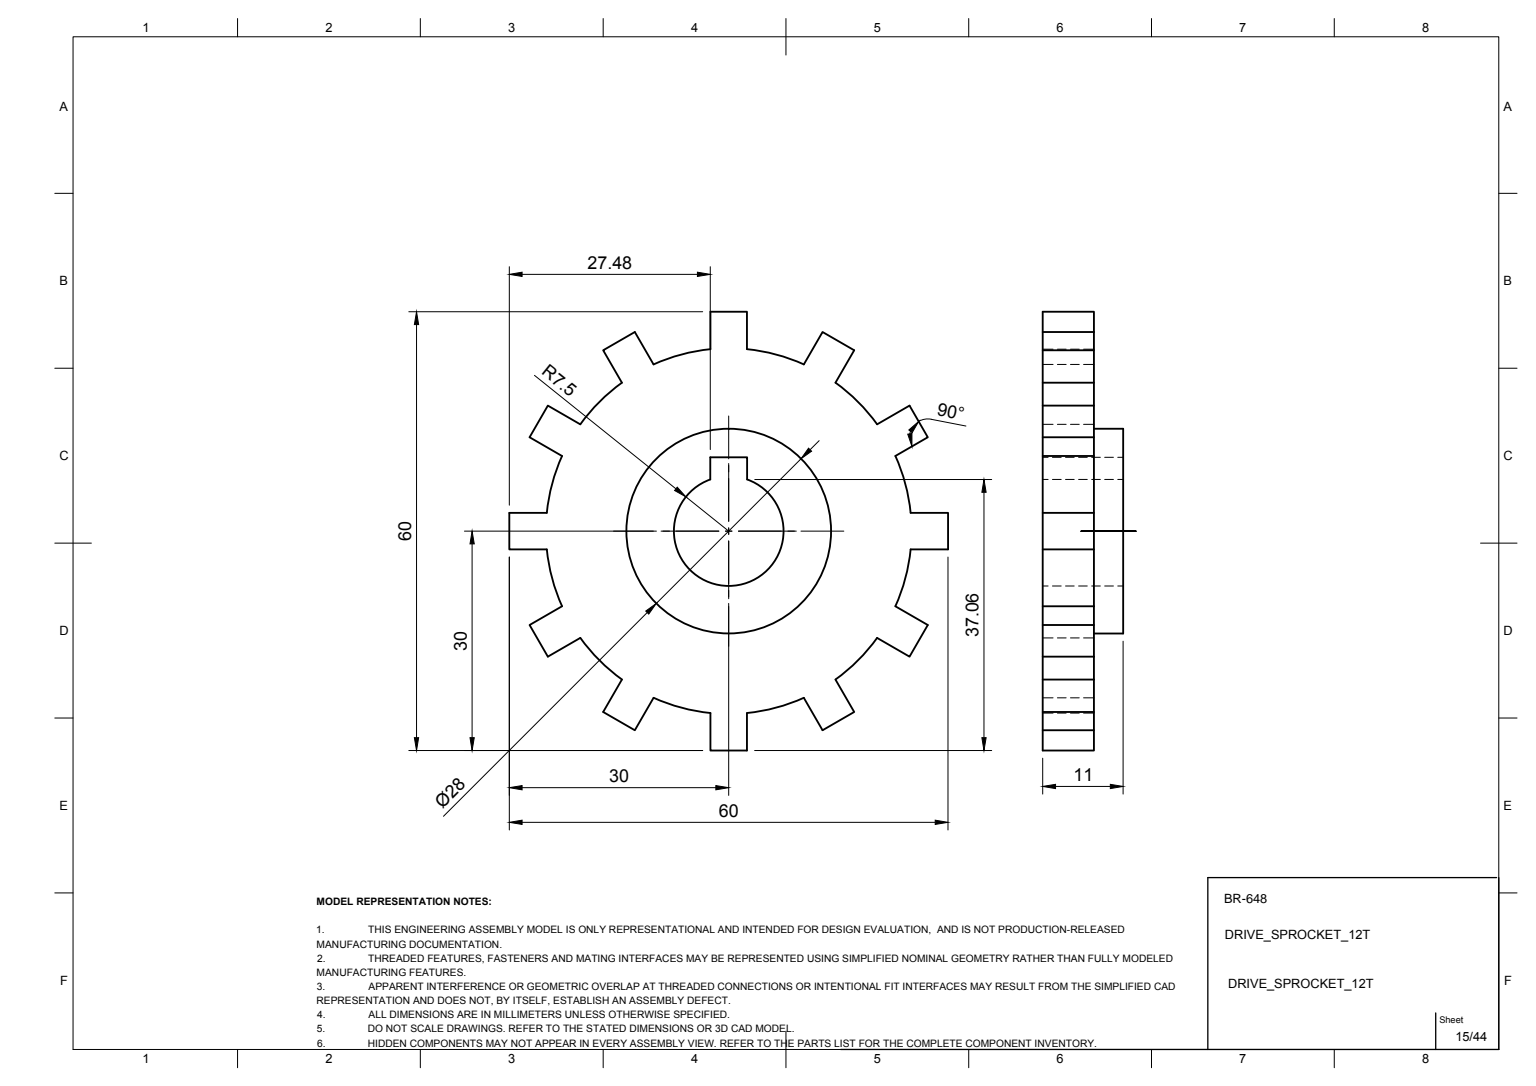
ISO-10303-21;
HEADER;
FILE_DESCRIPTION((''),'2;1');
FILE_NAME('DRIVE_SPROCKET_12T.step','2026-10-01T22:05:39-07:00',(''),(''),'','','');
FILE_SCHEMA (('AUTOMOTIVE_DESIGN { 1 0 10303 214 3 1 1 }'));
ENDSEC;
DATA;
#10=MECHANICAL_DESIGN_GEOMETRIC_PRESENTATION_REPRESENTATION('',(#615),#24628);
#531=SHAPE_REPRESENTATION_RELATIONSHIP('SRR','None',#24803,#573) ;
#573=ADVANCED_BREP_SHAPE_REPRESENTATION('',(#655),#24593) ;
#615=STYLED_ITEM('',(#25030),#655) ;
#655=MANIFOLD_SOLID_BREP('DRIVE_SPROCKET_12T',#13126) ;
#849=FACE_BOUND('',#4084,.T.) ;
#850=FACE_BOUND('',#4092,.T.) ;
#851=FACE_BOUND('',#4138,.T.) ;
#1160=LINE('',#20713,#1996) ;
#1161=LINE('',#20715,#1997) ;
#1162=LINE('',#20717,#1998) ;
#1163=LINE('',#20718,#1999) ;
#1164=LINE('',#20722,#2000) ;
#1165=LINE('',#20724,#2001) ;
#1166=LINE('',#20726,#2002) ;
#1167=LINE('',#20727,#2003) ;
#1168=LINE('',#20729,#2004) ;
#1169=LINE('',#20730,#2005) ;
#1170=LINE('',#20740,#2006) ;
#1171=LINE('',#20742,#2007) ;
#1172=LINE('',#20744,#2008) ;
#1173=LINE('',#20745,#2009) ;
#1174=LINE('',#20749,#2010) ;
#1175=LINE('',#20751,#2011) ;
#1176=LINE('',#20753,#2012) ;
#1177=LINE('',#20754,#2013) ;
#1178=LINE('',#20756,#2014) ;
#1179=LINE('',#20757,#2015) ;
#1180=LINE('',#20762,#2016) ;
#1181=LINE('',#20768,#2017) ;
#1182=LINE('',#20772,#2018) ;
#1183=LINE('',#20774,#2019) ;
#1184=LINE('',#20776,#2020) ;
#1185=LINE('',#20780,#2021) ;
#1186=LINE('',#20782,#2022) ;
#1187=LINE('',#20784,#2023) ;
#1188=LINE('',#20788,#2024) ;
#1189=LINE('',#20790,#2025) ;
#1190=LINE('',#20792,#2026) ;
#1191=LINE('',#20796,#2027) ;
#1192=LINE('',#20798,#2028) ;
#1193=LINE('',#20800,#2029) ;
#1194=LINE('',#20804,#2030) ;
#1195=LINE('',#20806,#2031) ;
#1196=LINE('',#20808,#2032) ;
#1197=LINE('',#20812,#2033) ;
#1198=LINE('',#20814,#2034) ;
#1199=LINE('',#20816,#2035) ;
#1200=LINE('',#20820,#2036) ;
#1201=LINE('',#20822,#2037) ;
#1202=LINE('',#20824,#2038) ;
#1203=LINE('',#20828,#2039) ;
#1204=LINE('',#20830,#2040) ;
#1205=LINE('',#20832,#2041) ;
#1206=LINE('',#20836,#2042) ;
#1207=LINE('',#20838,#2043) ;
#1208=LINE('',#20840,#2044) ;
#1209=LINE('',#20844,#2045) ;
#1210=LINE('',#20846,#2046) ;
#1211=LINE('',#20848,#2047) ;
#1212=LINE('',#20852,#2048) ;
#1213=LINE('',#20854,#2049) ;
#1214=LINE('',#20855,#2050) ;
#1215=LINE('',#20858,#2051) ;
#1216=LINE('',#20859,#2052) ;
#1217=LINE('',#20862,#2053) ;
#1218=LINE('',#20864,#2054) ;
#1219=LINE('',#20865,#2055) ;
#1220=LINE('',#20867,#2056) ;
#1221=LINE('',#20871,#2057) ;
#1222=LINE('',#20874,#2058) ;
#1223=LINE('',#20876,#2059) ;
#1224=LINE('',#20877,#2060) ;
#1225=LINE('',#20880,#2061) ;
#1226=LINE('',#20881,#2062) ;
#1227=LINE('',#20883,#2063) ;
#1228=LINE('',#20887,#2064) ;
#1229=LINE('',#20890,#2065) ;
#1230=LINE('',#20891,#2066) ;
#1231=LINE('',#20894,#2067) ;
#1232=LINE('',#20896,#2068) ;
#1233=LINE('',#20897,#2069) ;
#1234=LINE('',#20899,#2070) ;
#1235=LINE('',#20903,#2071) ;
#1236=LINE('',#20906,#2072) ;
#1237=LINE('',#20908,#2073) ;
#1238=LINE('',#20909,#2074) ;
#1239=LINE('',#20912,#2075) ;
#1240=LINE('',#20913,#2076) ;
#1241=LINE('',#20915,#2077) ;
#1242=LINE('',#20919,#2078) ;
#1243=LINE('',#20922,#2079) ;
#1244=LINE('',#20923,#2080) ;
#1245=LINE('',#20926,#2081) ;
#1246=LINE('',#20928,#2082) ;
#1247=LINE('',#20929,#2083) ;
#1248=LINE('',#20931,#2084) ;
#1249=LINE('',#20935,#2085) ;
#1250=LINE('',#20938,#2086) ;
#1251=LINE('',#20940,#2087) ;
#1252=LINE('',#20941,#2088) ;
#1253=LINE('',#20944,#2089) ;
#1254=LINE('',#20945,#2090) ;
#1255=LINE('',#20947,#2091) ;
#1256=LINE('',#20951,#2092) ;
#1257=LINE('',#20954,#2093) ;
#1258=LINE('',#20955,#2094) ;
#1259=LINE('',#20958,#2095) ;
#1260=LINE('',#20960,#2096) ;
#1261=LINE('',#20961,#2097) ;
#1262=LINE('',#20963,#2098) ;
#1263=LINE('',#20967,#2099) ;
#1264=LINE('',#20970,#2100) ;
#1265=LINE('',#20972,#2101) ;
#1266=LINE('',#20973,#2102) ;
#1267=LINE('',#20976,#2103) ;
#1268=LINE('',#20977,#2104) ;
#1269=LINE('',#20979,#2105) ;
#1270=LINE('',#20983,#2106) ;
#1271=LINE('',#20986,#2107) ;
#1272=LINE('',#20987,#2108) ;
#1273=LINE('',#20990,#2109) ;
#1274=LINE('',#20992,#2110) ;
#1275=LINE('',#20993,#2111) ;
#1276=LINE('',#20995,#2112) ;
#1277=LINE('',#20999,#2113) ;
#1278=LINE('',#21002,#2114) ;
#1279=LINE('',#21004,#2115) ;
#1280=LINE('',#21005,#2116) ;
#1281=LINE('',#21008,#2117) ;
#1282=LINE('',#21009,#2118) ;
#1283=LINE('',#21011,#2119) ;
#1284=LINE('',#21015,#2120) ;
#1285=LINE('',#21018,#2121) ;
#1286=LINE('',#21019,#2122) ;
#1287=LINE('',#21022,#2123) ;
#1288=LINE('',#21023,#2124) ;
#1289=LINE('',#21025,#2125) ;
#1290=LINE('',#21029,#2126) ;
#1996=VECTOR('',#16479,1.) ;
#1997=VECTOR('',#16480,1.) ;
#1998=VECTOR('',#16481,1.) ;
#1999=VECTOR('',#16482,1.) ;
#2000=VECTOR('',#16485,1.) ;
#2001=VECTOR('',#16486,1.) ;
#2002=VECTOR('',#16487,1.) ;
#2003=VECTOR('',#16488,1.) ;
#2004=VECTOR('',#16491,1.) ;
#2005=VECTOR('',#16492,1.) ;
#2006=VECTOR('',#16505,1.) ;
#2007=VECTOR('',#16506,1.) ;
#2008=VECTOR('',#16507,1.) ;
#2009=VECTOR('',#16508,1.) ;
#2010=VECTOR('',#16511,1.) ;
#2011=VECTOR('',#16512,1.) ;
#2012=VECTOR('',#16513,1.) ;
#2013=VECTOR('',#16514,1.) ;
#2014=VECTOR('',#16517,1.) ;
#2015=VECTOR('',#16518,1.) ;
#2016=VECTOR('',#16523,1.) ;
#2017=VECTOR('',#16530,1.) ;
#2018=VECTOR('',#16535,1.) ;
#2019=VECTOR('',#16536,1.) ;
#2020=VECTOR('',#16537,1.) ;
#2021=VECTOR('',#16540,1.) ;
#2022=VECTOR('',#16541,1.) ;
#2023=VECTOR('',#16542,1.) ;
#2024=VECTOR('',#16545,1.) ;
#2025=VECTOR('',#16546,1.) ;
#2026=VECTOR('',#16547,1.) ;
#2027=VECTOR('',#16550,1.) ;
#2028=VECTOR('',#16551,1.) ;
#2029=VECTOR('',#16552,1.) ;
#2030=VECTOR('',#16555,1.) ;
#2031=VECTOR('',#16556,1.) ;
#2032=VECTOR('',#16557,1.) ;
#2033=VECTOR('',#16560,1.) ;
#2034=VECTOR('',#16561,1.) ;
#2035=VECTOR('',#16562,1.) ;
#2036=VECTOR('',#16565,1.) ;
#2037=VECTOR('',#16566,1.) ;
#2038=VECTOR('',#16567,1.) ;
#2039=VECTOR('',#16570,1.) ;
#2040=VECTOR('',#16571,1.) ;
#2041=VECTOR('',#16572,1.) ;
#2042=VECTOR('',#16575,1.) ;
#2043=VECTOR('',#16576,1.) ;
#2044=VECTOR('',#16577,1.) ;
#2045=VECTOR('',#16580,1.) ;
#2046=VECTOR('',#16581,1.) ;
#2047=VECTOR('',#16582,1.) ;
#2048=VECTOR('',#16585,1.) ;
#2049=VECTOR('',#16586,1.) ;
#2050=VECTOR('',#16587,1.) ;
#2051=VECTOR('',#16590,1.) ;
#2052=VECTOR('',#16591,1.) ;
#2053=VECTOR('',#16594,1.) ;
#2054=VECTOR('',#16595,1.) ;
#2055=VECTOR('',#16596,1.) ;
#2056=VECTOR('',#16599,1.) ;
#2057=VECTOR('',#16604,1.) ;
#2058=VECTOR('',#16607,1.) ;
#2059=VECTOR('',#16608,1.) ;
#2060=VECTOR('',#16609,1.) ;
#2061=VECTOR('',#16612,1.) ;
#2062=VECTOR('',#16613,1.) ;
#2063=VECTOR('',#16616,1.) ;
#2064=VECTOR('',#16621,1.) ;
#2065=VECTOR('',#16624,1.) ;
#2066=VECTOR('',#16625,1.) ;
#2067=VECTOR('',#16628,1.) ;
#2068=VECTOR('',#16629,1.) ;
#2069=VECTOR('',#16630,1.) ;
#2070=VECTOR('',#16633,1.) ;
#2071=VECTOR('',#16638,1.) ;
#2072=VECTOR('',#16641,1.) ;
#2073=VECTOR('',#16642,1.) ;
#2074=VECTOR('',#16643,1.) ;
#2075=VECTOR('',#16646,1.) ;
#2076=VECTOR('',#16647,1.) ;
#2077=VECTOR('',#16650,1.) ;
#2078=VECTOR('',#16655,1.) ;
#2079=VECTOR('',#16658,1.) ;
#2080=VECTOR('',#16659,1.) ;
#2081=VECTOR('',#16662,1.) ;
#2082=VECTOR('',#16663,1.) ;
#2083=VECTOR('',#16664,1.) ;
#2084=VECTOR('',#16667,1.) ;
#2085=VECTOR('',#16672,1.) ;
#2086=VECTOR('',#16675,1.) ;
#2087=VECTOR('',#16676,1.) ;
#2088=VECTOR('',#16677,1.) ;
#2089=VECTOR('',#16680,1.) ;
#2090=VECTOR('',#16681,1.) ;
#2091=VECTOR('',#16684,1.) ;
#2092=VECTOR('',#16689,1.) ;
#2093=VECTOR('',#16692,1.) ;
#2094=VECTOR('',#16693,1.) ;
#2095=VECTOR('',#16696,1.) ;
#2096=VECTOR('',#16697,1.) ;
#2097=VECTOR('',#16698,1.) ;
#2098=VECTOR('',#16701,1.) ;
#2099=VECTOR('',#16706,1.) ;
#2100=VECTOR('',#16709,1.) ;
#2101=VECTOR('',#16710,1.) ;
#2102=VECTOR('',#16711,1.) ;
#2103=VECTOR('',#16714,1.) ;
#2104=VECTOR('',#16715,1.) ;
#2105=VECTOR('',#16718,1.) ;
#2106=VECTOR('',#16723,1.) ;
#2107=VECTOR('',#16726,1.) ;
#2108=VECTOR('',#16727,1.) ;
#2109=VECTOR('',#16730,1.) ;
#2110=VECTOR('',#16731,1.) ;
#2111=VECTOR('',#16732,1.) ;
#2112=VECTOR('',#16735,1.) ;
#2113=VECTOR('',#16740,1.) ;
#2114=VECTOR('',#16743,1.) ;
#2115=VECTOR('',#16744,1.) ;
#2116=VECTOR('',#16745,1.) ;
#2117=VECTOR('',#16748,1.) ;
#2118=VECTOR('',#16749,1.) ;
#2119=VECTOR('',#16752,1.) ;
#2120=VECTOR('',#16757,1.) ;
#2121=VECTOR('',#16760,1.) ;
#2122=VECTOR('',#16761,1.) ;
#2123=VECTOR('',#16764,1.) ;
#2124=VECTOR('',#16765,1.) ;
#2125=VECTOR('',#16768,1.) ;
#2126=VECTOR('',#16773,1.4) ;
#2790=CYLINDRICAL_SURFACE('',#14122,0.75) ;
#2791=CYLINDRICAL_SURFACE('',#14127,2.5) ;
#2792=CYLINDRICAL_SURFACE('',#14130,2.5) ;
#2793=CYLINDRICAL_SURFACE('',#14147,2.5) ;
#2794=CYLINDRICAL_SURFACE('',#14152,2.5) ;
#2795=CYLINDRICAL_SURFACE('',#14157,2.5) ;
#2796=CYLINDRICAL_SURFACE('',#14162,2.5) ;
#2797=CYLINDRICAL_SURFACE('',#14167,2.5) ;
#2798=CYLINDRICAL_SURFACE('',#14172,2.5) ;
#2799=CYLINDRICAL_SURFACE('',#14177,2.5) ;
#2800=CYLINDRICAL_SURFACE('',#14182,2.5) ;
#2801=CYLINDRICAL_SURFACE('',#14187,2.5) ;
#2802=CYLINDRICAL_SURFACE('',#14192,2.5) ;
#2803=CYLINDRICAL_SURFACE('',#14197,1.4) ;
#3150=FACE_OUTER_BOUND('',#4080,.T.) ;
#3151=FACE_OUTER_BOUND('',#4081,.T.) ;
#3152=FACE_OUTER_BOUND('',#4082,.T.) ;
#3153=FACE_OUTER_BOUND('',#4083,.T.) ;
#3154=FACE_OUTER_BOUND('',#4085,.T.) ;
#3155=FACE_OUTER_BOUND('',#4086,.T.) ;
#3156=FACE_OUTER_BOUND('',#4087,.T.) ;
#3157=FACE_OUTER_BOUND('',#4088,.T.) ;
#3158=FACE_OUTER_BOUND('',#4089,.T.) ;
#3159=FACE_OUTER_BOUND('',#4090,.T.) ;
#3160=FACE_OUTER_BOUND('',#4091,.T.) ;
#3161=FACE_OUTER_BOUND('',#4093,.T.) ;
#3162=FACE_OUTER_BOUND('',#4094,.T.) ;
#3163=FACE_OUTER_BOUND('',#4095,.T.) ;
#3164=FACE_OUTER_BOUND('',#4096,.T.) ;
#3165=FACE_OUTER_BOUND('',#4097,.T.) ;
#3166=FACE_OUTER_BOUND('',#4098,.T.) ;
#3167=FACE_OUTER_BOUND('',#4099,.T.) ;
#3168=FACE_OUTER_BOUND('',#4100,.T.) ;
#3169=FACE_OUTER_BOUND('',#4101,.T.) ;
#3170=FACE_OUTER_BOUND('',#4102,.T.) ;
#3171=FACE_OUTER_BOUND('',#4103,.T.) ;
#3172=FACE_OUTER_BOUND('',#4104,.T.) ;
#3173=FACE_OUTER_BOUND('',#4105,.T.) ;
#3174=FACE_OUTER_BOUND('',#4106,.T.) ;
#3175=FACE_OUTER_BOUND('',#4107,.T.) ;
#3176=FACE_OUTER_BOUND('',#4108,.T.) ;
#3177=FACE_OUTER_BOUND('',#4109,.T.) ;
#3178=FACE_OUTER_BOUND('',#4110,.T.) ;
#3179=FACE_OUTER_BOUND('',#4111,.T.) ;
#3180=FACE_OUTER_BOUND('',#4112,.T.) ;
#3181=FACE_OUTER_BOUND('',#4113,.T.) ;
#3182=FACE_OUTER_BOUND('',#4114,.T.) ;
#3183=FACE_OUTER_BOUND('',#4115,.T.) ;
#3184=FACE_OUTER_BOUND('',#4116,.T.) ;
#3185=FACE_OUTER_BOUND('',#4117,.T.) ;
#3186=FACE_OUTER_BOUND('',#4118,.T.) ;
#3187=FACE_OUTER_BOUND('',#4119,.T.) ;
#3188=FACE_OUTER_BOUND('',#4120,.T.) ;
#3189=FACE_OUTER_BOUND('',#4121,.T.) ;
#3190=FACE_OUTER_BOUND('',#4122,.T.) ;
#3191=FACE_OUTER_BOUND('',#4123,.T.) ;
#3192=FACE_OUTER_BOUND('',#4124,.T.) ;
#3193=FACE_OUTER_BOUND('',#4125,.T.) ;
#3194=FACE_OUTER_BOUND('',#4126,.T.) ;
#3195=FACE_OUTER_BOUND('',#4127,.T.) ;
#3196=FACE_OUTER_BOUND('',#4128,.T.) ;
#3197=FACE_OUTER_BOUND('',#4129,.T.) ;
#3198=FACE_OUTER_BOUND('',#4130,.T.) ;
#3199=FACE_OUTER_BOUND('',#4131,.T.) ;
#3200=FACE_OUTER_BOUND('',#4132,.T.) ;
#3201=FACE_OUTER_BOUND('',#4133,.T.) ;
#3202=FACE_OUTER_BOUND('',#4134,.T.) ;
#3203=FACE_OUTER_BOUND('',#4135,.T.) ;
#3204=FACE_OUTER_BOUND('',#4136,.T.) ;
#3205=FACE_OUTER_BOUND('',#4137,.T.) ;
#4080=EDGE_LOOP('',(#9321,#9322,#9323,#9324)) ;
#4081=EDGE_LOOP('',(#9325,#9326,#9327,#9328)) ;
#4082=EDGE_LOOP('',(#9329,#9330,#9331,#9332)) ;
#4083=EDGE_LOOP('',(#9333)) ;
#4084=EDGE_LOOP('',(#9334,#9335,#9336,#9337)) ;
#4085=EDGE_LOOP('',(#9338,#9339,#9340,#9341)) ;
#4086=EDGE_LOOP('',(#9342,#9343,#9344,#9345)) ;
#4087=EDGE_LOOP('',(#9346,#9347,#9348,#9349)) ;
#4088=EDGE_LOOP('',(#9350,#9351,#9352,#9353)) ;
#4089=EDGE_LOOP('',(#9354,#9355,#9356,#9357)) ;
#4090=EDGE_LOOP('',(#9358,#9359,#9360,#9361)) ;
#4091=EDGE_LOOP('',(#9362,#9363,#9364,#9365,#9366,#9367,#9368,#9369,#9370,
#9371,#9372,#9373,#9374,#9375,#9376,#9377,#9378,#9379,#9380,#9381,#9382,
#9383,#9384,#9385,#9386,#9387,#9388,#9389,#9390,#9391,#9392,#9393,#9394,
#9395,#9396,#9397,#9398,#9399,#9400,#9401,#9402,#9403,#9404,#9405,#9406,
#9407,#9408,#9409)) ;
#4092=EDGE_LOOP('',(#9410,#9411,#9412,#9413)) ;
#4093=EDGE_LOOP('',(#9414,#9415,#9416,#9417)) ;
#4094=EDGE_LOOP('',(#9418,#9419,#9420,#9421)) ;
#4095=EDGE_LOOP('',(#9422,#9423,#9424,#9425)) ;
#4096=EDGE_LOOP('',(#9426,#9427,#9428,#9429)) ;
#4097=EDGE_LOOP('',(#9430,#9431,#9432,#9433)) ;
#4098=EDGE_LOOP('',(#9434,#9435,#9436,#9437)) ;
#4099=EDGE_LOOP('',(#9438,#9439,#9440,#9441)) ;
#4100=EDGE_LOOP('',(#9442,#9443,#9444,#9445)) ;
#4101=EDGE_LOOP('',(#9446,#9447,#9448,#9449)) ;
#4102=EDGE_LOOP('',(#9450,#9451,#9452,#9453)) ;
#4103=EDGE_LOOP('',(#9454,#9455,#9456,#9457)) ;
#4104=EDGE_LOOP('',(#9458,#9459,#9460,#9461)) ;
#4105=EDGE_LOOP('',(#9462,#9463,#9464,#9465)) ;
#4106=EDGE_LOOP('',(#9466,#9467,#9468,#9469)) ;
#4107=EDGE_LOOP('',(#9470,#9471,#9472,#9473)) ;
#4108=EDGE_LOOP('',(#9474,#9475,#9476,#9477)) ;
#4109=EDGE_LOOP('',(#9478,#9479,#9480,#9481)) ;
#4110=EDGE_LOOP('',(#9482,#9483,#9484,#9485)) ;
#4111=EDGE_LOOP('',(#9486,#9487,#9488,#9489)) ;
#4112=EDGE_LOOP('',(#9490,#9491,#9492,#9493)) ;
#4113=EDGE_LOOP('',(#9494,#9495,#9496,#9497)) ;
#4114=EDGE_LOOP('',(#9498,#9499,#9500,#9501)) ;
#4115=EDGE_LOOP('',(#9502,#9503,#9504,#9505)) ;
#4116=EDGE_LOOP('',(#9506,#9507,#9508,#9509)) ;
#4117=EDGE_LOOP('',(#9510,#9511,#9512,#9513)) ;
#4118=EDGE_LOOP('',(#9514,#9515,#9516,#9517)) ;
#4119=EDGE_LOOP('',(#9518,#9519,#9520,#9521)) ;
#4120=EDGE_LOOP('',(#9522,#9523,#9524,#9525)) ;
#4121=EDGE_LOOP('',(#9526,#9527,#9528,#9529)) ;
#4122=EDGE_LOOP('',(#9530,#9531,#9532,#9533)) ;
#4123=EDGE_LOOP('',(#9534,#9535,#9536,#9537)) ;
#4124=EDGE_LOOP('',(#9538,#9539,#9540,#9541)) ;
#4125=EDGE_LOOP('',(#9542,#9543,#9544,#9545)) ;
#4126=EDGE_LOOP('',(#9546,#9547,#9548,#9549)) ;
#4127=EDGE_LOOP('',(#9550,#9551,#9552,#9553)) ;
#4128=EDGE_LOOP('',(#9554,#9555,#9556,#9557)) ;
#4129=EDGE_LOOP('',(#9558,#9559,#9560,#9561)) ;
#4130=EDGE_LOOP('',(#9562,#9563,#9564,#9565)) ;
#4131=EDGE_LOOP('',(#9566,#9567,#9568,#9569)) ;
#4132=EDGE_LOOP('',(#9570,#9571,#9572,#9573)) ;
#4133=EDGE_LOOP('',(#9574,#9575,#9576,#9577)) ;
#4134=EDGE_LOOP('',(#9578,#9579,#9580,#9581)) ;
#4135=EDGE_LOOP('',(#9582,#9583,#9584,#9585)) ;
#4136=EDGE_LOOP('',(#9586,#9587,#9588,#9589)) ;
#4137=EDGE_LOOP('',(#9590,#9591,#9592,#9593,#9594,#9595,#9596,#9597,#9598,
#9599,#9600,#9601,#9602,#9603,#9604,#9605,#9606,#9607,#9608,#9609,#9610,
#9611,#9612,#9613,#9614,#9615,#9616,#9617,#9618,#9619,#9620,#9621,#9622,
#9623,#9624,#9625,#9626,#9627,#9628,#9629,#9630,#9631,#9632,#9633,#9634,
#9635,#9636,#9637)) ;
#4138=EDGE_LOOP('',(#9638)) ;
#5004=CIRCLE('',#14120,1.4) ;
#5005=CIRCLE('',#14121,0.75) ;
#5006=CIRCLE('',#14123,0.75) ;
#5007=CIRCLE('',#14128,2.5) ;
#5008=CIRCLE('',#14129,2.5) ;
#5009=CIRCLE('',#14131,2.5) ;
#5010=CIRCLE('',#14132,2.5) ;
#5011=CIRCLE('',#14134,2.5) ;
#5012=CIRCLE('',#14135,2.5) ;
#5013=CIRCLE('',#14136,2.5) ;
#5014=CIRCLE('',#14137,2.5) ;
#5015=CIRCLE('',#14138,2.5) ;
#5016=CIRCLE('',#14139,2.5) ;
#5017=CIRCLE('',#14140,2.5) ;
#5018=CIRCLE('',#14141,2.5) ;
#5019=CIRCLE('',#14142,2.5) ;
#5020=CIRCLE('',#14143,2.5) ;
#5021=CIRCLE('',#14148,2.5) ;
#5022=CIRCLE('',#14153,2.5) ;
#5023=CIRCLE('',#14158,2.5) ;
#5024=CIRCLE('',#14163,2.5) ;
#5025=CIRCLE('',#14168,2.5) ;
#5026=CIRCLE('',#14173,2.5) ;
#5027=CIRCLE('',#14178,2.5) ;
#5028=CIRCLE('',#14183,2.5) ;
#5029=CIRCLE('',#14188,2.5) ;
#5030=CIRCLE('',#14193,2.5) ;
#5031=CIRCLE('',#14198,1.4) ;
#5815=VERTEX_POINT('',#20711) ;
#5816=VERTEX_POINT('',#20712) ;
#5817=VERTEX_POINT('',#20714) ;
#5818=VERTEX_POINT('',#20716) ;
#5819=VERTEX_POINT('',#20720) ;
#5820=VERTEX_POINT('',#20721) ;
#5821=VERTEX_POINT('',#20723) ;
#5822=VERTEX_POINT('',#20725) ;
#5823=VERTEX_POINT('',#20732) ;
#5824=VERTEX_POINT('',#20738) ;
#5825=VERTEX_POINT('',#20739) ;
#5826=VERTEX_POINT('',#20741) ;
#5827=VERTEX_POINT('',#20743) ;
#5828=VERTEX_POINT('',#20747) ;
#5829=VERTEX_POINT('',#20748) ;
#5830=VERTEX_POINT('',#20750) ;
#5831=VERTEX_POINT('',#20752) ;
#5832=VERTEX_POINT('',#20759) ;
#5833=VERTEX_POINT('',#20761) ;
#5834=VERTEX_POINT('',#20765) ;
#5835=VERTEX_POINT('',#20767) ;
#5836=VERTEX_POINT('',#20771) ;
#5837=VERTEX_POINT('',#20773) ;
#5838=VERTEX_POINT('',#20775) ;
#5839=VERTEX_POINT('',#20777) ;
#5840=VERTEX_POINT('',#20779) ;
#5841=VERTEX_POINT('',#20781) ;
#5842=VERTEX_POINT('',#20783) ;
#5843=VERTEX_POINT('',#20785) ;
#5844=VERTEX_POINT('',#20787) ;
#5845=VERTEX_POINT('',#20789) ;
#5846=VERTEX_POINT('',#20791) ;
#5847=VERTEX_POINT('',#20793) ;
#5848=VERTEX_POINT('',#20795) ;
#5849=VERTEX_POINT('',#20797) ;
#5850=VERTEX_POINT('',#20799) ;
#5851=VERTEX_POINT('',#20801) ;
#5852=VERTEX_POINT('',#20803) ;
#5853=VERTEX_POINT('',#20805) ;
#5854=VERTEX_POINT('',#20807) ;
#5855=VERTEX_POINT('',#20809) ;
#5856=VERTEX_POINT('',#20811) ;
#5857=VERTEX_POINT('',#20813) ;
#5858=VERTEX_POINT('',#20815) ;
#5859=VERTEX_POINT('',#20817) ;
#5860=VERTEX_POINT('',#20819) ;
#5861=VERTEX_POINT('',#20821) ;
#5862=VERTEX_POINT('',#20823) ;
#5863=VERTEX_POINT('',#20825) ;
#5864=VERTEX_POINT('',#20827) ;
#5865=VERTEX_POINT('',#20829) ;
#5866=VERTEX_POINT('',#20831) ;
#5867=VERTEX_POINT('',#20833) ;
#5868=VERTEX_POINT('',#20835) ;
#5869=VERTEX_POINT('',#20837) ;
#5870=VERTEX_POINT('',#20839) ;
#5871=VERTEX_POINT('',#20841) ;
#5872=VERTEX_POINT('',#20843) ;
#5873=VERTEX_POINT('',#20845) ;
#5874=VERTEX_POINT('',#20847) ;
#5875=VERTEX_POINT('',#20849) ;
#5876=VERTEX_POINT('',#20851) ;
#5877=VERTEX_POINT('',#20853) ;
#5878=VERTEX_POINT('',#20857) ;
#5879=VERTEX_POINT('',#20861) ;
#5880=VERTEX_POINT('',#20863) ;
#5881=VERTEX_POINT('',#20869) ;
#5882=VERTEX_POINT('',#20873) ;
#5883=VERTEX_POINT('',#20875) ;
#5884=VERTEX_POINT('',#20879) ;
#5885=VERTEX_POINT('',#20885) ;
#5886=VERTEX_POINT('',#20889) ;
#5887=VERTEX_POINT('',#20893) ;
#5888=VERTEX_POINT('',#20895) ;
#5889=VERTEX_POINT('',#20901) ;
#5890=VERTEX_POINT('',#20905) ;
#5891=VERTEX_POINT('',#20907) ;
#5892=VERTEX_POINT('',#20911) ;
#5893=VERTEX_POINT('',#20917) ;
#5894=VERTEX_POINT('',#20921) ;
#5895=VERTEX_POINT('',#20925) ;
#5896=VERTEX_POINT('',#20927) ;
#5897=VERTEX_POINT('',#20933) ;
#5898=VERTEX_POINT('',#20937) ;
#5899=VERTEX_POINT('',#20939) ;
#5900=VERTEX_POINT('',#20943) ;
#5901=VERTEX_POINT('',#20949) ;
#5902=VERTEX_POINT('',#20953) ;
#5903=VERTEX_POINT('',#20957) ;
#5904=VERTEX_POINT('',#20959) ;
#5905=VERTEX_POINT('',#20965) ;
#5906=VERTEX_POINT('',#20969) ;
#5907=VERTEX_POINT('',#20971) ;
#5908=VERTEX_POINT('',#20975) ;
#5909=VERTEX_POINT('',#20981) ;
#5910=VERTEX_POINT('',#20985) ;
#5911=VERTEX_POINT('',#20989) ;
#5912=VERTEX_POINT('',#20991) ;
#5913=VERTEX_POINT('',#20997) ;
#5914=VERTEX_POINT('',#21001) ;
#5915=VERTEX_POINT('',#21003) ;
#5916=VERTEX_POINT('',#21007) ;
#5917=VERTEX_POINT('',#21013) ;
#5918=VERTEX_POINT('',#21017) ;
#5919=VERTEX_POINT('',#21021) ;
#5920=VERTEX_POINT('',#21027) ;
#7150=EDGE_CURVE('',#5815,#5816,#1160,.T.) ;
#7151=EDGE_CURVE('',#5817,#5815,#1161,.T.) ;
#7152=EDGE_CURVE('',#5818,#5817,#1162,.T.) ;
#7153=EDGE_CURVE('',#5816,#5818,#1163,.T.) ;
#7154=EDGE_CURVE('',#5819,#5820,#1164,.T.) ;
#7155=EDGE_CURVE('',#5821,#5819,#1165,.T.) ;
#7156=EDGE_CURVE('',#5822,#5821,#1166,.T.) ;
#7157=EDGE_CURVE('',#5820,#5822,#1167,.T.) ;
#7158=EDGE_CURVE('',#5820,#5815,#1168,.T.) ;
#7159=EDGE_CURVE('',#5817,#5822,#1169,.T.) ;
#7160=EDGE_CURVE('',#5823,#5823,#5004,.T.) ;
#7161=EDGE_CURVE('',#5821,#5818,#5005,.T.) ;
#7162=EDGE_CURVE('',#5816,#5819,#5006,.T.) ;
#7163=EDGE_CURVE('',#5824,#5825,#1170,.T.) ;
#7164=EDGE_CURVE('',#5824,#5826,#1171,.T.) ;
#7165=EDGE_CURVE('',#5826,#5827,#1172,.T.) ;
#7166=EDGE_CURVE('',#5827,#5825,#1173,.T.) ;
#7167=EDGE_CURVE('',#5828,#5829,#1174,.T.) ;
#7168=EDGE_CURVE('',#5828,#5830,#1175,.T.) ;
#7169=EDGE_CURVE('',#5830,#5831,#1176,.T.) ;
#7170=EDGE_CURVE('',#5831,#5829,#1177,.T.) ;
#7171=EDGE_CURVE('',#5830,#5827,#1178,.T.) ;
#7172=EDGE_CURVE('',#5831,#5826,#1179,.T.) ;
#7173=EDGE_CURVE('',#5832,#5825,#5007,.T.) ;
#7174=EDGE_CURVE('',#5832,#5833,#1180,.T.) ;
#7175=EDGE_CURVE('',#5824,#5833,#5008,.T.) ;
#7176=EDGE_CURVE('',#5834,#5829,#5009,.T.) ;
#7177=EDGE_CURVE('',#5834,#5835,#1181,.T.) ;
#7178=EDGE_CURVE('',#5828,#5835,#5010,.T.) ;
#7179=EDGE_CURVE('',#5836,#5833,#1182,.T.) ;
#7180=EDGE_CURVE('',#5836,#5837,#1183,.T.) ;
#7181=EDGE_CURVE('',#5838,#5837,#1184,.T.) ;
#7182=EDGE_CURVE('',#5838,#5839,#5011,.T.) ;
#7183=EDGE_CURVE('',#5840,#5839,#1185,.T.) ;
#7184=EDGE_CURVE('',#5840,#5841,#1186,.T.) ;
#7185=EDGE_CURVE('',#5842,#5841,#1187,.T.) ;
#7186=EDGE_CURVE('',#5842,#5843,#5012,.T.) ;
#7187=EDGE_CURVE('',#5844,#5843,#1188,.T.) ;
#7188=EDGE_CURVE('',#5844,#5845,#1189,.T.) ;
#7189=EDGE_CURVE('',#5846,#5845,#1190,.T.) ;
#7190=EDGE_CURVE('',#5846,#5847,#5013,.T.) ;
#7191=EDGE_CURVE('',#5848,#5847,#1191,.T.) ;
#7192=EDGE_CURVE('',#5848,#5849,#1192,.T.) ;
#7193=EDGE_CURVE('',#5850,#5849,#1193,.T.) ;
#7194=EDGE_CURVE('',#5850,#5851,#5014,.T.) ;
#7195=EDGE_CURVE('',#5852,#5851,#1194,.T.) ;
#7196=EDGE_CURVE('',#5852,#5853,#1195,.T.) ;
#7197=EDGE_CURVE('',#5854,#5853,#1196,.T.) ;
#7198=EDGE_CURVE('',#5854,#5855,#5015,.T.) ;
#7199=EDGE_CURVE('',#5856,#5855,#1197,.T.) ;
#7200=EDGE_CURVE('',#5856,#5857,#1198,.T.) ;
#7201=EDGE_CURVE('',#5858,#5857,#1199,.T.) ;
#7202=EDGE_CURVE('',#5858,#5859,#5016,.T.) ;
#7203=EDGE_CURVE('',#5860,#5859,#1200,.T.) ;
#7204=EDGE_CURVE('',#5860,#5861,#1201,.T.) ;
#7205=EDGE_CURVE('',#5862,#5861,#1202,.T.) ;
#7206=EDGE_CURVE('',#5862,#5863,#5017,.T.) ;
#7207=EDGE_CURVE('',#5864,#5863,#1203,.T.) ;
#7208=EDGE_CURVE('',#5864,#5865,#1204,.T.) ;
#7209=EDGE_CURVE('',#5866,#5865,#1205,.T.) ;
#7210=EDGE_CURVE('',#5866,#5867,#5018,.T.) ;
#7211=EDGE_CURVE('',#5868,#5867,#1206,.T.) ;
#7212=EDGE_CURVE('',#5868,#5869,#1207,.T.) ;
#7213=EDGE_CURVE('',#5870,#5869,#1208,.T.) ;
#7214=EDGE_CURVE('',#5870,#5871,#5019,.T.) ;
#7215=EDGE_CURVE('',#5872,#5871,#1209,.T.) ;
#7216=EDGE_CURVE('',#5872,#5873,#1210,.T.) ;
#7217=EDGE_CURVE('',#5874,#5873,#1211,.T.) ;
#7218=EDGE_CURVE('',#5874,#5875,#5020,.T.) ;
#7219=EDGE_CURVE('',#5876,#5875,#1212,.T.) ;
#7220=EDGE_CURVE('',#5876,#5877,#1213,.T.) ;
#7221=EDGE_CURVE('',#5834,#5877,#1214,.T.) ;
#7222=EDGE_CURVE('',#5832,#5878,#1215,.T.) ;
#7223=EDGE_CURVE('',#5878,#5836,#1216,.T.) ;
#7224=EDGE_CURVE('',#5838,#5879,#1217,.T.) ;
#7225=EDGE_CURVE('',#5837,#5880,#1218,.T.) ;
#7226=EDGE_CURVE('',#5880,#5879,#1219,.T.) ;
#7227=EDGE_CURVE('',#5878,#5880,#1220,.T.) ;
#7228=EDGE_CURVE('',#5881,#5879,#5021,.T.) ;
#7229=EDGE_CURVE('',#5881,#5839,#1221,.T.) ;
#7230=EDGE_CURVE('',#5842,#5882,#1222,.T.) ;
#7231=EDGE_CURVE('',#5841,#5883,#1223,.T.) ;
#7232=EDGE_CURVE('',#5883,#5882,#1224,.T.) ;
#7233=EDGE_CURVE('',#5881,#5884,#1225,.T.) ;
#7234=EDGE_CURVE('',#5884,#5840,#1226,.T.) ;
#7235=EDGE_CURVE('',#5884,#5883,#1227,.T.) ;
#7236=EDGE_CURVE('',#5885,#5882,#5022,.T.) ;
#7237=EDGE_CURVE('',#5885,#5843,#1228,.T.) ;
#7238=EDGE_CURVE('',#5885,#5886,#1229,.T.) ;
#7239=EDGE_CURVE('',#5886,#5844,#1230,.T.) ;
#7240=EDGE_CURVE('',#5846,#5887,#1231,.T.) ;
#7241=EDGE_CURVE('',#5845,#5888,#1232,.T.) ;
#7242=EDGE_CURVE('',#5888,#5887,#1233,.T.) ;
#7243=EDGE_CURVE('',#5886,#5888,#1234,.T.) ;
#7244=EDGE_CURVE('',#5889,#5887,#5023,.T.) ;
#7245=EDGE_CURVE('',#5889,#5847,#1235,.T.) ;
#7246=EDGE_CURVE('',#5850,#5890,#1236,.T.) ;
#7247=EDGE_CURVE('',#5849,#5891,#1237,.T.) ;
#7248=EDGE_CURVE('',#5891,#5890,#1238,.T.) ;
#7249=EDGE_CURVE('',#5889,#5892,#1239,.T.) ;
#7250=EDGE_CURVE('',#5892,#5848,#1240,.T.) ;
#7251=EDGE_CURVE('',#5892,#5891,#1241,.T.) ;
#7252=EDGE_CURVE('',#5893,#5890,#5024,.T.) ;
#7253=EDGE_CURVE('',#5893,#5851,#1242,.T.) ;
#7254=EDGE_CURVE('',#5893,#5894,#1243,.T.) ;
#7255=EDGE_CURVE('',#5894,#5852,#1244,.T.) ;
#7256=EDGE_CURVE('',#5854,#5895,#1245,.T.) ;
#7257=EDGE_CURVE('',#5853,#5896,#1246,.T.) ;
#7258=EDGE_CURVE('',#5896,#5895,#1247,.T.) ;
#7259=EDGE_CURVE('',#5894,#5896,#1248,.T.) ;
#7260=EDGE_CURVE('',#5897,#5895,#5025,.T.) ;
#7261=EDGE_CURVE('',#5897,#5855,#1249,.T.) ;
#7262=EDGE_CURVE('',#5858,#5898,#1250,.T.) ;
#7263=EDGE_CURVE('',#5857,#5899,#1251,.T.) ;
#7264=EDGE_CURVE('',#5899,#5898,#1252,.T.) ;
#7265=EDGE_CURVE('',#5897,#5900,#1253,.T.) ;
#7266=EDGE_CURVE('',#5900,#5856,#1254,.T.) ;
#7267=EDGE_CURVE('',#5900,#5899,#1255,.T.) ;
#7268=EDGE_CURVE('',#5901,#5898,#5026,.T.) ;
#7269=EDGE_CURVE('',#5901,#5859,#1256,.T.) ;
#7270=EDGE_CURVE('',#5901,#5902,#1257,.T.) ;
#7271=EDGE_CURVE('',#5902,#5860,#1258,.T.) ;
#7272=EDGE_CURVE('',#5862,#5903,#1259,.T.) ;
#7273=EDGE_CURVE('',#5861,#5904,#1260,.T.) ;
#7274=EDGE_CURVE('',#5904,#5903,#1261,.T.) ;
#7275=EDGE_CURVE('',#5902,#5904,#1262,.T.) ;
#7276=EDGE_CURVE('',#5905,#5903,#5027,.T.) ;
#7277=EDGE_CURVE('',#5905,#5863,#1263,.T.) ;
#7278=EDGE_CURVE('',#5866,#5906,#1264,.T.) ;
#7279=EDGE_CURVE('',#5865,#5907,#1265,.T.) ;
#7280=EDGE_CURVE('',#5907,#5906,#1266,.T.) ;
#7281=EDGE_CURVE('',#5905,#5908,#1267,.T.) ;
#7282=EDGE_CURVE('',#5908,#5864,#1268,.T.) ;
#7283=EDGE_CURVE('',#5908,#5907,#1269,.T.) ;
#7284=EDGE_CURVE('',#5909,#5906,#5028,.T.) ;
#7285=EDGE_CURVE('',#5909,#5867,#1270,.T.) ;
#7286=EDGE_CURVE('',#5909,#5910,#1271,.T.) ;
#7287=EDGE_CURVE('',#5910,#5868,#1272,.T.) ;
#7288=EDGE_CURVE('',#5870,#5911,#1273,.T.) ;
#7289=EDGE_CURVE('',#5869,#5912,#1274,.T.) ;
#7290=EDGE_CURVE('',#5912,#5911,#1275,.T.) ;
#7291=EDGE_CURVE('',#5910,#5912,#1276,.T.) ;
#7292=EDGE_CURVE('',#5913,#5911,#5029,.T.) ;
#7293=EDGE_CURVE('',#5913,#5871,#1277,.T.) ;
#7294=EDGE_CURVE('',#5874,#5914,#1278,.T.) ;
#7295=EDGE_CURVE('',#5873,#5915,#1279,.T.) ;
#7296=EDGE_CURVE('',#5915,#5914,#1280,.T.) ;
#7297=EDGE_CURVE('',#5913,#5916,#1281,.T.) ;
#7298=EDGE_CURVE('',#5916,#5872,#1282,.T.) ;
#7299=EDGE_CURVE('',#5916,#5915,#1283,.T.) ;
#7300=EDGE_CURVE('',#5917,#5914,#5030,.T.) ;
#7301=EDGE_CURVE('',#5917,#5875,#1284,.T.) ;
#7302=EDGE_CURVE('',#5917,#5918,#1285,.T.) ;
#7303=EDGE_CURVE('',#5918,#5876,#1286,.T.) ;
#7304=EDGE_CURVE('',#5877,#5919,#1287,.T.) ;
#7305=EDGE_CURVE('',#5919,#5835,#1288,.T.) ;
#7306=EDGE_CURVE('',#5918,#5919,#1289,.T.) ;
#7307=EDGE_CURVE('',#5920,#5920,#5031,.T.) ;
#7308=EDGE_CURVE('',#5920,#5823,#1290,.T.) ;
#9321=ORIENTED_EDGE('',*,*,#7150,.F.) ;
#9322=ORIENTED_EDGE('',*,*,#7151,.F.) ;
#9323=ORIENTED_EDGE('',*,*,#7152,.F.) ;
#9324=ORIENTED_EDGE('',*,*,#7153,.F.) ;
#9325=ORIENTED_EDGE('',*,*,#7154,.F.) ;
#9326=ORIENTED_EDGE('',*,*,#7155,.F.) ;
#9327=ORIENTED_EDGE('',*,*,#7156,.F.) ;
#9328=ORIENTED_EDGE('',*,*,#7157,.F.) ;
#9329=ORIENTED_EDGE('',*,*,#7158,.F.) ;
#9330=ORIENTED_EDGE('',*,*,#7157,.T.) ;
#9331=ORIENTED_EDGE('',*,*,#7159,.F.) ;
#9332=ORIENTED_EDGE('',*,*,#7151,.T.) ;
#9333=ORIENTED_EDGE('',*,*,#7160,.T.) ;
#9334=ORIENTED_EDGE('',*,*,#7152,.T.) ;
#9335=ORIENTED_EDGE('',*,*,#7159,.T.) ;
#9336=ORIENTED_EDGE('',*,*,#7156,.T.) ;
#9337=ORIENTED_EDGE('',*,*,#7161,.T.) ;
#9338=ORIENTED_EDGE('',*,*,#7153,.T.) ;
#9339=ORIENTED_EDGE('',*,*,#7161,.F.) ;
#9340=ORIENTED_EDGE('',*,*,#7155,.T.) ;
#9341=ORIENTED_EDGE('',*,*,#7162,.F.) ;
#9342=ORIENTED_EDGE('',*,*,#7163,.F.) ;
#9343=ORIENTED_EDGE('',*,*,#7164,.T.) ;
#9344=ORIENTED_EDGE('',*,*,#7165,.T.) ;
#9345=ORIENTED_EDGE('',*,*,#7166,.T.) ;
#9346=ORIENTED_EDGE('',*,*,#7167,.F.) ;
#9347=ORIENTED_EDGE('',*,*,#7168,.T.) ;
#9348=ORIENTED_EDGE('',*,*,#7169,.T.) ;
#9349=ORIENTED_EDGE('',*,*,#7170,.T.) ;
#9350=ORIENTED_EDGE('',*,*,#7171,.T.) ;
#9351=ORIENTED_EDGE('',*,*,#7165,.F.) ;
#9352=ORIENTED_EDGE('',*,*,#7172,.F.) ;
#9353=ORIENTED_EDGE('',*,*,#7169,.F.) ;
#9354=ORIENTED_EDGE('',*,*,#7163,.T.) ;
#9355=ORIENTED_EDGE('',*,*,#7173,.F.) ;
#9356=ORIENTED_EDGE('',*,*,#7174,.T.) ;
#9357=ORIENTED_EDGE('',*,*,#7175,.F.) ;
#9358=ORIENTED_EDGE('',*,*,#7167,.T.) ;
#9359=ORIENTED_EDGE('',*,*,#7176,.F.) ;
#9360=ORIENTED_EDGE('',*,*,#7177,.T.) ;
#9361=ORIENTED_EDGE('',*,*,#7178,.F.) ;
#9362=ORIENTED_EDGE('',*,*,#7175,.T.) ;
#9363=ORIENTED_EDGE('',*,*,#7179,.F.) ;
#9364=ORIENTED_EDGE('',*,*,#7180,.T.) ;
#9365=ORIENTED_EDGE('',*,*,#7181,.F.) ;
#9366=ORIENTED_EDGE('',*,*,#7182,.T.) ;
#9367=ORIENTED_EDGE('',*,*,#7183,.F.) ;
#9368=ORIENTED_EDGE('',*,*,#7184,.T.) ;
#9369=ORIENTED_EDGE('',*,*,#7185,.F.) ;
#9370=ORIENTED_EDGE('',*,*,#7186,.T.) ;
#9371=ORIENTED_EDGE('',*,*,#7187,.F.) ;
#9372=ORIENTED_EDGE('',*,*,#7188,.T.) ;
#9373=ORIENTED_EDGE('',*,*,#7189,.F.) ;
#9374=ORIENTED_EDGE('',*,*,#7190,.T.) ;
#9375=ORIENTED_EDGE('',*,*,#7191,.F.) ;
#9376=ORIENTED_EDGE('',*,*,#7192,.T.) ;
#9377=ORIENTED_EDGE('',*,*,#7193,.F.) ;
#9378=ORIENTED_EDGE('',*,*,#7194,.T.) ;
#9379=ORIENTED_EDGE('',*,*,#7195,.F.) ;
#9380=ORIENTED_EDGE('',*,*,#7196,.T.) ;
#9381=ORIENTED_EDGE('',*,*,#7197,.F.) ;
#9382=ORIENTED_EDGE('',*,*,#7198,.T.) ;
#9383=ORIENTED_EDGE('',*,*,#7199,.F.) ;
#9384=ORIENTED_EDGE('',*,*,#7200,.T.) ;
#9385=ORIENTED_EDGE('',*,*,#7201,.F.) ;
#9386=ORIENTED_EDGE('',*,*,#7202,.T.) ;
#9387=ORIENTED_EDGE('',*,*,#7203,.F.) ;
#9388=ORIENTED_EDGE('',*,*,#7204,.T.) ;
#9389=ORIENTED_EDGE('',*,*,#7205,.F.) ;
#9390=ORIENTED_EDGE('',*,*,#7206,.T.) ;
#9391=ORIENTED_EDGE('',*,*,#7207,.F.) ;
#9392=ORIENTED_EDGE('',*,*,#7208,.T.) ;
#9393=ORIENTED_EDGE('',*,*,#7209,.F.) ;
#9394=ORIENTED_EDGE('',*,*,#7210,.T.) ;
#9395=ORIENTED_EDGE('',*,*,#7211,.F.) ;
#9396=ORIENTED_EDGE('',*,*,#7212,.T.) ;
#9397=ORIENTED_EDGE('',*,*,#7213,.F.) ;
#9398=ORIENTED_EDGE('',*,*,#7214,.T.) ;
#9399=ORIENTED_EDGE('',*,*,#7215,.F.) ;
#9400=ORIENTED_EDGE('',*,*,#7216,.T.) ;
#9401=ORIENTED_EDGE('',*,*,#7217,.F.) ;
#9402=ORIENTED_EDGE('',*,*,#7218,.T.) ;
#9403=ORIENTED_EDGE('',*,*,#7219,.F.) ;
#9404=ORIENTED_EDGE('',*,*,#7220,.T.) ;
#9405=ORIENTED_EDGE('',*,*,#7221,.F.) ;
#9406=ORIENTED_EDGE('',*,*,#7176,.T.) ;
#9407=ORIENTED_EDGE('',*,*,#7170,.F.) ;
#9408=ORIENTED_EDGE('',*,*,#7172,.T.) ;
#9409=ORIENTED_EDGE('',*,*,#7164,.F.) ;
#9410=ORIENTED_EDGE('',*,*,#7150,.T.) ;
#9411=ORIENTED_EDGE('',*,*,#7162,.T.) ;
#9412=ORIENTED_EDGE('',*,*,#7154,.T.) ;
#9413=ORIENTED_EDGE('',*,*,#7158,.T.) ;
#9414=ORIENTED_EDGE('',*,*,#7174,.F.) ;
#9415=ORIENTED_EDGE('',*,*,#7222,.T.) ;
#9416=ORIENTED_EDGE('',*,*,#7223,.T.) ;
#9417=ORIENTED_EDGE('',*,*,#7179,.T.) ;
#9418=ORIENTED_EDGE('',*,*,#7224,.F.) ;
#9419=ORIENTED_EDGE('',*,*,#7181,.T.) ;
#9420=ORIENTED_EDGE('',*,*,#7225,.T.) ;
#9421=ORIENTED_EDGE('',*,*,#7226,.T.) ;
#9422=ORIENTED_EDGE('',*,*,#7227,.T.) ;
#9423=ORIENTED_EDGE('',*,*,#7225,.F.) ;
#9424=ORIENTED_EDGE('',*,*,#7180,.F.) ;
#9425=ORIENTED_EDGE('',*,*,#7223,.F.) ;
#9426=ORIENTED_EDGE('',*,*,#7224,.T.) ;
#9427=ORIENTED_EDGE('',*,*,#7228,.F.) ;
#9428=ORIENTED_EDGE('',*,*,#7229,.T.) ;
#9429=ORIENTED_EDGE('',*,*,#7182,.F.) ;
#9430=ORIENTED_EDGE('',*,*,#7230,.F.) ;
#9431=ORIENTED_EDGE('',*,*,#7185,.T.) ;
#9432=ORIENTED_EDGE('',*,*,#7231,.T.) ;
#9433=ORIENTED_EDGE('',*,*,#7232,.T.) ;
#9434=ORIENTED_EDGE('',*,*,#7229,.F.) ;
#9435=ORIENTED_EDGE('',*,*,#7233,.T.) ;
#9436=ORIENTED_EDGE('',*,*,#7234,.T.) ;
#9437=ORIENTED_EDGE('',*,*,#7183,.T.) ;
#9438=ORIENTED_EDGE('',*,*,#7235,.T.) ;
#9439=ORIENTED_EDGE('',*,*,#7231,.F.) ;
#9440=ORIENTED_EDGE('',*,*,#7184,.F.) ;
#9441=ORIENTED_EDGE('',*,*,#7234,.F.) ;
#9442=ORIENTED_EDGE('',*,*,#7230,.T.) ;
#9443=ORIENTED_EDGE('',*,*,#7236,.F.) ;
#9444=ORIENTED_EDGE('',*,*,#7237,.T.) ;
#9445=ORIENTED_EDGE('',*,*,#7186,.F.) ;
#9446=ORIENTED_EDGE('',*,*,#7237,.F.) ;
#9447=ORIENTED_EDGE('',*,*,#7238,.T.) ;
#9448=ORIENTED_EDGE('',*,*,#7239,.T.) ;
#9449=ORIENTED_EDGE('',*,*,#7187,.T.) ;
#9450=ORIENTED_EDGE('',*,*,#7240,.F.) ;
#9451=ORIENTED_EDGE('',*,*,#7189,.T.) ;
#9452=ORIENTED_EDGE('',*,*,#7241,.T.) ;
#9453=ORIENTED_EDGE('',*,*,#7242,.T.) ;
#9454=ORIENTED_EDGE('',*,*,#7243,.T.) ;
#9455=ORIENTED_EDGE('',*,*,#7241,.F.) ;
#9456=ORIENTED_EDGE('',*,*,#7188,.F.) ;
#9457=ORIENTED_EDGE('',*,*,#7239,.F.) ;
#9458=ORIENTED_EDGE('',*,*,#7240,.T.) ;
#9459=ORIENTED_EDGE('',*,*,#7244,.F.) ;
#9460=ORIENTED_EDGE('',*,*,#7245,.T.) ;
#9461=ORIENTED_EDGE('',*,*,#7190,.F.) ;
#9462=ORIENTED_EDGE('',*,*,#7246,.F.) ;
#9463=ORIENTED_EDGE('',*,*,#7193,.T.) ;
#9464=ORIENTED_EDGE('',*,*,#7247,.T.) ;
#9465=ORIENTED_EDGE('',*,*,#7248,.T.) ;
#9466=ORIENTED_EDGE('',*,*,#7245,.F.) ;
#9467=ORIENTED_EDGE('',*,*,#7249,.T.) ;
#9468=ORIENTED_EDGE('',*,*,#7250,.T.) ;
#9469=ORIENTED_EDGE('',*,*,#7191,.T.) ;
#9470=ORIENTED_EDGE('',*,*,#7251,.T.) ;
#9471=ORIENTED_EDGE('',*,*,#7247,.F.) ;
#9472=ORIENTED_EDGE('',*,*,#7192,.F.) ;
#9473=ORIENTED_EDGE('',*,*,#7250,.F.) ;
#9474=ORIENTED_EDGE('',*,*,#7246,.T.) ;
#9475=ORIENTED_EDGE('',*,*,#7252,.F.) ;
#9476=ORIENTED_EDGE('',*,*,#7253,.T.) ;
#9477=ORIENTED_EDGE('',*,*,#7194,.F.) ;
#9478=ORIENTED_EDGE('',*,*,#7253,.F.) ;
#9479=ORIENTED_EDGE('',*,*,#7254,.T.) ;
#9480=ORIENTED_EDGE('',*,*,#7255,.T.) ;
#9481=ORIENTED_EDGE('',*,*,#7195,.T.) ;
#9482=ORIENTED_EDGE('',*,*,#7256,.F.) ;
#9483=ORIENTED_EDGE('',*,*,#7197,.T.) ;
#9484=ORIENTED_EDGE('',*,*,#7257,.T.) ;
#9485=ORIENTED_EDGE('',*,*,#7258,.T.) ;
#9486=ORIENTED_EDGE('',*,*,#7259,.T.) ;
#9487=ORIENTED_EDGE('',*,*,#7257,.F.) ;
#9488=ORIENTED_EDGE('',*,*,#7196,.F.) ;
#9489=ORIENTED_EDGE('',*,*,#7255,.F.) ;
#9490=ORIENTED_EDGE('',*,*,#7256,.T.) ;
#9491=ORIENTED_EDGE('',*,*,#7260,.F.) ;
#9492=ORIENTED_EDGE('',*,*,#7261,.T.) ;
#9493=ORIENTED_EDGE('',*,*,#7198,.F.) ;
#9494=ORIENTED_EDGE('',*,*,#7262,.F.) ;
#9495=ORIENTED_EDGE('',*,*,#7201,.T.) ;
#9496=ORIENTED_EDGE('',*,*,#7263,.T.) ;
#9497=ORIENTED_EDGE('',*,*,#7264,.T.) ;
#9498=ORIENTED_EDGE('',*,*,#7261,.F.) ;
#9499=ORIENTED_EDGE('',*,*,#7265,.T.) ;
#9500=ORIENTED_EDGE('',*,*,#7266,.T.) ;
#9501=ORIENTED_EDGE('',*,*,#7199,.T.) ;
#9502=ORIENTED_EDGE('',*,*,#7267,.T.) ;
#9503=ORIENTED_EDGE('',*,*,#7263,.F.) ;
#9504=ORIENTED_EDGE('',*,*,#7200,.F.) ;
#9505=ORIENTED_EDGE('',*,*,#7266,.F.) ;
#9506=ORIENTED_EDGE('',*,*,#7262,.T.) ;
#9507=ORIENTED_EDGE('',*,*,#7268,.F.) ;
#9508=ORIENTED_EDGE('',*,*,#7269,.T.) ;
#9509=ORIENTED_EDGE('',*,*,#7202,.F.) ;
#9510=ORIENTED_EDGE('',*,*,#7269,.F.) ;
#9511=ORIENTED_EDGE('',*,*,#7270,.T.) ;
#9512=ORIENTED_EDGE('',*,*,#7271,.T.) ;
#9513=ORIENTED_EDGE('',*,*,#7203,.T.) ;
#9514=ORIENTED_EDGE('',*,*,#7272,.F.) ;
#9515=ORIENTED_EDGE('',*,*,#7205,.T.) ;
#9516=ORIENTED_EDGE('',*,*,#7273,.T.) ;
#9517=ORIENTED_EDGE('',*,*,#7274,.T.) ;
#9518=ORIENTED_EDGE('',*,*,#7275,.T.) ;
#9519=ORIENTED_EDGE('',*,*,#7273,.F.) ;
#9520=ORIENTED_EDGE('',*,*,#7204,.F.) ;
#9521=ORIENTED_EDGE('',*,*,#7271,.F.) ;
#9522=ORIENTED_EDGE('',*,*,#7272,.T.) ;
#9523=ORIENTED_EDGE('',*,*,#7276,.F.) ;
#9524=ORIENTED_EDGE('',*,*,#7277,.T.) ;
#9525=ORIENTED_EDGE('',*,*,#7206,.F.) ;
#9526=ORIENTED_EDGE('',*,*,#7278,.F.) ;
#9527=ORIENTED_EDGE('',*,*,#7209,.T.) ;
#9528=ORIENTED_EDGE('',*,*,#7279,.T.) ;
#9529=ORIENTED_EDGE('',*,*,#7280,.T.) ;
#9530=ORIENTED_EDGE('',*,*,#7277,.F.) ;
#9531=ORIENTED_EDGE('',*,*,#7281,.T.) ;
#9532=ORIENTED_EDGE('',*,*,#7282,.T.) ;
#9533=ORIENTED_EDGE('',*,*,#7207,.T.) ;
#9534=ORIENTED_EDGE('',*,*,#7283,.T.) ;
#9535=ORIENTED_EDGE('',*,*,#7279,.F.) ;
#9536=ORIENTED_EDGE('',*,*,#7208,.F.) ;
#9537=ORIENTED_EDGE('',*,*,#7282,.F.) ;
#9538=ORIENTED_EDGE('',*,*,#7278,.T.) ;
#9539=ORIENTED_EDGE('',*,*,#7284,.F.) ;
#9540=ORIENTED_EDGE('',*,*,#7285,.T.) ;
#9541=ORIENTED_EDGE('',*,*,#7210,.F.) ;
#9542=ORIENTED_EDGE('',*,*,#7285,.F.) ;
#9543=ORIENTED_EDGE('',*,*,#7286,.T.) ;
#9544=ORIENTED_EDGE('',*,*,#7287,.T.) ;
#9545=ORIENTED_EDGE('',*,*,#7211,.T.) ;
#9546=ORIENTED_EDGE('',*,*,#7288,.F.) ;
#9547=ORIENTED_EDGE('',*,*,#7213,.T.) ;
#9548=ORIENTED_EDGE('',*,*,#7289,.T.) ;
#9549=ORIENTED_EDGE('',*,*,#7290,.T.) ;
#9550=ORIENTED_EDGE('',*,*,#7291,.T.) ;
#9551=ORIENTED_EDGE('',*,*,#7289,.F.) ;
#9552=ORIENTED_EDGE('',*,*,#7212,.F.) ;
#9553=ORIENTED_EDGE('',*,*,#7287,.F.) ;
#9554=ORIENTED_EDGE('',*,*,#7288,.T.) ;
#9555=ORIENTED_EDGE('',*,*,#7292,.F.) ;
#9556=ORIENTED_EDGE('',*,*,#7293,.T.) ;
#9557=ORIENTED_EDGE('',*,*,#7214,.F.) ;
#9558=ORIENTED_EDGE('',*,*,#7294,.F.) ;
#9559=ORIENTED_EDGE('',*,*,#7217,.T.) ;
#9560=ORIENTED_EDGE('',*,*,#7295,.T.) ;
#9561=ORIENTED_EDGE('',*,*,#7296,.T.) ;
#9562=ORIENTED_EDGE('',*,*,#7293,.F.) ;
#9563=ORIENTED_EDGE('',*,*,#7297,.T.) ;
#9564=ORIENTED_EDGE('',*,*,#7298,.T.) ;
#9565=ORIENTED_EDGE('',*,*,#7215,.T.) ;
#9566=ORIENTED_EDGE('',*,*,#7299,.T.) ;
#9567=ORIENTED_EDGE('',*,*,#7295,.F.) ;
#9568=ORIENTED_EDGE('',*,*,#7216,.F.) ;
#9569=ORIENTED_EDGE('',*,*,#7298,.F.) ;
#9570=ORIENTED_EDGE('',*,*,#7294,.T.) ;
#9571=ORIENTED_EDGE('',*,*,#7300,.F.) ;
#9572=ORIENTED_EDGE('',*,*,#7301,.T.) ;
#9573=ORIENTED_EDGE('',*,*,#7218,.F.) ;
#9574=ORIENTED_EDGE('',*,*,#7301,.F.) ;
#9575=ORIENTED_EDGE('',*,*,#7302,.T.) ;
#9576=ORIENTED_EDGE('',*,*,#7303,.T.) ;
#9577=ORIENTED_EDGE('',*,*,#7219,.T.) ;
#9578=ORIENTED_EDGE('',*,*,#7177,.F.) ;
#9579=ORIENTED_EDGE('',*,*,#7221,.T.) ;
#9580=ORIENTED_EDGE('',*,*,#7304,.T.) ;
#9581=ORIENTED_EDGE('',*,*,#7305,.T.) ;
#9582=ORIENTED_EDGE('',*,*,#7306,.T.) ;
#9583=ORIENTED_EDGE('',*,*,#7304,.F.) ;
#9584=ORIENTED_EDGE('',*,*,#7220,.F.) ;
#9585=ORIENTED_EDGE('',*,*,#7303,.F.) ;
#9586=ORIENTED_EDGE('',*,*,#7307,.F.) ;
#9587=ORIENTED_EDGE('',*,*,#7308,.T.) ;
#9588=ORIENTED_EDGE('',*,*,#7160,.F.) ;
#9589=ORIENTED_EDGE('',*,*,#7308,.F.) ;
#9590=ORIENTED_EDGE('',*,*,#7178,.T.) ;
#9591=ORIENTED_EDGE('',*,*,#7305,.F.) ;
#9592=ORIENTED_EDGE('',*,*,#7306,.F.) ;
#9593=ORIENTED_EDGE('',*,*,#7302,.F.) ;
#9594=ORIENTED_EDGE('',*,*,#7300,.T.) ;
#9595=ORIENTED_EDGE('',*,*,#7296,.F.) ;
#9596=ORIENTED_EDGE('',*,*,#7299,.F.) ;
#9597=ORIENTED_EDGE('',*,*,#7297,.F.) ;
#9598=ORIENTED_EDGE('',*,*,#7292,.T.) ;
#9599=ORIENTED_EDGE('',*,*,#7290,.F.) ;
#9600=ORIENTED_EDGE('',*,*,#7291,.F.) ;
#9601=ORIENTED_EDGE('',*,*,#7286,.F.) ;
#9602=ORIENTED_EDGE('',*,*,#7284,.T.) ;
#9603=ORIENTED_EDGE('',*,*,#7280,.F.) ;
#9604=ORIENTED_EDGE('',*,*,#7283,.F.) ;
#9605=ORIENTED_EDGE('',*,*,#7281,.F.) ;
#9606=ORIENTED_EDGE('',*,*,#7276,.T.) ;
#9607=ORIENTED_EDGE('',*,*,#7274,.F.) ;
#9608=ORIENTED_EDGE('',*,*,#7275,.F.) ;
#9609=ORIENTED_EDGE('',*,*,#7270,.F.) ;
#9610=ORIENTED_EDGE('',*,*,#7268,.T.) ;
#9611=ORIENTED_EDGE('',*,*,#7264,.F.) ;
#9612=ORIENTED_EDGE('',*,*,#7267,.F.) ;
#9613=ORIENTED_EDGE('',*,*,#7265,.F.) ;
#9614=ORIENTED_EDGE('',*,*,#7260,.T.) ;
#9615=ORIENTED_EDGE('',*,*,#7258,.F.) ;
#9616=ORIENTED_EDGE('',*,*,#7259,.F.) ;
#9617=ORIENTED_EDGE('',*,*,#7254,.F.) ;
#9618=ORIENTED_EDGE('',*,*,#7252,.T.) ;
#9619=ORIENTED_EDGE('',*,*,#7248,.F.) ;
#9620=ORIENTED_EDGE('',*,*,#7251,.F.) ;
#9621=ORIENTED_EDGE('',*,*,#7249,.F.) ;
#9622=ORIENTED_EDGE('',*,*,#7244,.T.) ;
#9623=ORIENTED_EDGE('',*,*,#7242,.F.) ;
#9624=ORIENTED_EDGE('',*,*,#7243,.F.) ;
#9625=ORIENTED_EDGE('',*,*,#7238,.F.) ;
#9626=ORIENTED_EDGE('',*,*,#7236,.T.) ;
#9627=ORIENTED_EDGE('',*,*,#7232,.F.) ;
#9628=ORIENTED_EDGE('',*,*,#7235,.F.) ;
#9629=ORIENTED_EDGE('',*,*,#7233,.F.) ;
#9630=ORIENTED_EDGE('',*,*,#7228,.T.) ;
#9631=ORIENTED_EDGE('',*,*,#7226,.F.) ;
#9632=ORIENTED_EDGE('',*,*,#7227,.F.) ;
#9633=ORIENTED_EDGE('',*,*,#7222,.F.) ;
#9634=ORIENTED_EDGE('',*,*,#7173,.T.) ;
#9635=ORIENTED_EDGE('',*,*,#7166,.F.) ;
#9636=ORIENTED_EDGE('',*,*,#7171,.F.) ;
#9637=ORIENTED_EDGE('',*,*,#7168,.F.) ;
#9638=ORIENTED_EDGE('',*,*,#7307,.T.) ;
#12076=PLANE('',#14116) ;
#12077=PLANE('',#14117) ;
#12078=PLANE('',#14118) ;
#12079=PLANE('',#14119) ;
#12080=PLANE('',#14124) ;
#12081=PLANE('',#14125) ;
#12082=PLANE('',#14126) ;
#12083=PLANE('',#14133) ;
#12084=PLANE('',#14144) ;
#12085=PLANE('',#14145) ;
#12086=PLANE('',#14146) ;
#12087=PLANE('',#14149) ;
#12088=PLANE('',#14150) ;
#12089=PLANE('',#14151) ;
#12090=PLANE('',#14154) ;
#12091=PLANE('',#14155) ;
#12092=PLANE('',#14156) ;
#12093=PLANE('',#14159) ;
#12094=PLANE('',#14160) ;
#12095=PLANE('',#14161) ;
#12096=PLANE('',#14164) ;
#12097=PLANE('',#14165) ;
#12098=PLANE('',#14166) ;
#12099=PLANE('',#14169) ;
#12100=PLANE('',#14170) ;
#12101=PLANE('',#14171) ;
#12102=PLANE('',#14174) ;
#12103=PLANE('',#14175) ;
#12104=PLANE('',#14176) ;
#12105=PLANE('',#14179) ;
#12106=PLANE('',#14180) ;
#12107=PLANE('',#14181) ;
#12108=PLANE('',#14184) ;
#12109=PLANE('',#14185) ;
#12110=PLANE('',#14186) ;
#12111=PLANE('',#14189) ;
#12112=PLANE('',#14190) ;
#12113=PLANE('',#14191) ;
#12114=PLANE('',#14194) ;
#12115=PLANE('',#14195) ;
#12116=PLANE('',#14196) ;
#12117=PLANE('',#14199) ;
#12545=ADVANCED_FACE('',(#3150),#12076,.F.) ;
#12546=ADVANCED_FACE('',(#3151),#12077,.T.) ;
#12547=ADVANCED_FACE('',(#3152),#12078,.T.) ;
#12548=ADVANCED_FACE('',(#3153,#849),#12079,.T.) ;
#12549=ADVANCED_FACE('',(#3154),#2790,.F.) ;
#12550=ADVANCED_FACE('',(#3155),#12080,.F.) ;
#12551=ADVANCED_FACE('',(#3156),#12081,.T.) ;
#12552=ADVANCED_FACE('',(#3157),#12082,.F.) ;
#12553=ADVANCED_FACE('',(#3158),#2791,.T.) ;
#12554=ADVANCED_FACE('',(#3159),#2792,.T.) ;
#12555=ADVANCED_FACE('',(#3160,#850),#12083,.T.) ;
#12556=ADVANCED_FACE('',(#3161),#12084,.T.) ;
#12557=ADVANCED_FACE('',(#3162),#12085,.F.) ;
#12558=ADVANCED_FACE('',(#3163),#12086,.F.) ;
#12559=ADVANCED_FACE('',(#3164),#2793,.T.) ;
#12560=ADVANCED_FACE('',(#3165),#12087,.F.) ;
#12561=ADVANCED_FACE('',(#3166),#12088,.T.) ;
#12562=ADVANCED_FACE('',(#3167),#12089,.F.) ;
#12563=ADVANCED_FACE('',(#3168),#2794,.T.) ;
#12564=ADVANCED_FACE('',(#3169),#12090,.T.) ;
#12565=ADVANCED_FACE('',(#3170),#12091,.F.) ;
#12566=ADVANCED_FACE('',(#3171),#12092,.F.) ;
#12567=ADVANCED_FACE('',(#3172),#2795,.T.) ;
#12568=ADVANCED_FACE('',(#3173),#12093,.F.) ;
#12569=ADVANCED_FACE('',(#3174),#12094,.T.) ;
#12570=ADVANCED_FACE('',(#3175),#12095,.F.) ;
#12571=ADVANCED_FACE('',(#3176),#2796,.T.) ;
#12572=ADVANCED_FACE('',(#3177),#12096,.T.) ;
#12573=ADVANCED_FACE('',(#3178),#12097,.F.) ;
#12574=ADVANCED_FACE('',(#3179),#12098,.F.) ;
#12575=ADVANCED_FACE('',(#3180),#2797,.T.) ;
#12576=ADVANCED_FACE('',(#3181),#12099,.F.) ;
#12577=ADVANCED_FACE('',(#3182),#12100,.T.) ;
#12578=ADVANCED_FACE('',(#3183),#12101,.F.) ;
#12579=ADVANCED_FACE('',(#3184),#2798,.T.) ;
#12580=ADVANCED_FACE('',(#3185),#12102,.T.) ;
#12581=ADVANCED_FACE('',(#3186),#12103,.F.) ;
#12582=ADVANCED_FACE('',(#3187),#12104,.F.) ;
#12583=ADVANCED_FACE('',(#3188),#2799,.T.) ;
#12584=ADVANCED_FACE('',(#3189),#12105,.F.) ;
#12585=ADVANCED_FACE('',(#3190),#12106,.T.) ;
#12586=ADVANCED_FACE('',(#3191),#12107,.F.) ;
#12587=ADVANCED_FACE('',(#3192),#2800,.T.) ;
#12588=ADVANCED_FACE('',(#3193),#12108,.T.) ;
#12589=ADVANCED_FACE('',(#3194),#12109,.F.) ;
#12590=ADVANCED_FACE('',(#3195),#12110,.F.) ;
#12591=ADVANCED_FACE('',(#3196),#2801,.T.) ;
#12592=ADVANCED_FACE('',(#3197),#12111,.F.) ;
#12593=ADVANCED_FACE('',(#3198),#12112,.T.) ;
#12594=ADVANCED_FACE('',(#3199),#12113,.F.) ;
#12595=ADVANCED_FACE('',(#3200),#2802,.T.) ;
#12596=ADVANCED_FACE('',(#3201),#12114,.T.) ;
#12597=ADVANCED_FACE('',(#3202),#12115,.F.) ;
#12598=ADVANCED_FACE('',(#3203),#12116,.F.) ;
#12599=ADVANCED_FACE('',(#3204),#2803,.T.) ;
#12600=ADVANCED_FACE('',(#3205,#851),#12117,.T.) ;
#13126=CLOSED_SHELL('',(#12545,#12546,#12547,#12548,#12549,#12550,#12551,
#12552,#12553,#12554,#12555,#12556,#12557,#12558,#12559,#12560,#12561,#12562,
#12563,#12564,#12565,#12566,#12567,#12568,#12569,#12570,#12571,#12572,#12573,
#12574,#12575,#12576,#12577,#12578,#12579,#12580,#12581,#12582,#12583,#12584,
#12585,#12586,#12587,#12588,#12589,#12590,#12591,#12592,#12593,#12594,#12595,
#12596,#12597,#12598,#12599,#12600)) ;
#14115=AXIS2_PLACEMENT_3D('',#20709,#16475,#16476) ;
#14116=AXIS2_PLACEMENT_3D('',#20710,#16477,#16478) ;
#14117=AXIS2_PLACEMENT_3D('',#20719,#16483,#16484) ;
#14118=AXIS2_PLACEMENT_3D('',#20728,#16489,#16490) ;
#14119=AXIS2_PLACEMENT_3D('',#20731,#16493,#16494) ;
#14120=AXIS2_PLACEMENT_3D('',#20733,#16495,#16496) ;
#14121=AXIS2_PLACEMENT_3D('',#20734,#16497,#16498) ;
#14122=AXIS2_PLACEMENT_3D('',#20735,#16499,#16500) ;
#14123=AXIS2_PLACEMENT_3D('',#20736,#16501,#16502) ;
#14124=AXIS2_PLACEMENT_3D('',#20737,#16503,#16504) ;
#14125=AXIS2_PLACEMENT_3D('',#20746,#16509,#16510) ;
#14126=AXIS2_PLACEMENT_3D('',#20755,#16515,#16516) ;
#14127=AXIS2_PLACEMENT_3D('',#20758,#16519,#16520) ;
#14128=AXIS2_PLACEMENT_3D('',#20760,#16521,#16522) ;
#14129=AXIS2_PLACEMENT_3D('',#20763,#16524,#16525) ;
#14130=AXIS2_PLACEMENT_3D('',#20764,#16526,#16527) ;
#14131=AXIS2_PLACEMENT_3D('',#20766,#16528,#16529) ;
#14132=AXIS2_PLACEMENT_3D('',#20769,#16531,#16532) ;
#14133=AXIS2_PLACEMENT_3D('',#20770,#16533,#16534) ;
#14134=AXIS2_PLACEMENT_3D('',#20778,#16538,#16539) ;
#14135=AXIS2_PLACEMENT_3D('',#20786,#16543,#16544) ;
#14136=AXIS2_PLACEMENT_3D('',#20794,#16548,#16549) ;
#14137=AXIS2_PLACEMENT_3D('',#20802,#16553,#16554) ;
#14138=AXIS2_PLACEMENT_3D('',#20810,#16558,#16559) ;
#14139=AXIS2_PLACEMENT_3D('',#20818,#16563,#16564) ;
#14140=AXIS2_PLACEMENT_3D('',#20826,#16568,#16569) ;
#14141=AXIS2_PLACEMENT_3D('',#20834,#16573,#16574) ;
#14142=AXIS2_PLACEMENT_3D('',#20842,#16578,#16579) ;
#14143=AXIS2_PLACEMENT_3D('',#20850,#16583,#16584) ;
#14144=AXIS2_PLACEMENT_3D('',#20856,#16588,#16589) ;
#14145=AXIS2_PLACEMENT_3D('',#20860,#16592,#16593) ;
#14146=AXIS2_PLACEMENT_3D('',#20866,#16597,#16598) ;
#14147=AXIS2_PLACEMENT_3D('',#20868,#16600,#16601) ;
#14148=AXIS2_PLACEMENT_3D('',#20870,#16602,#16603) ;
#14149=AXIS2_PLACEMENT_3D('',#20872,#16605,#16606) ;
#14150=AXIS2_PLACEMENT_3D('',#20878,#16610,#16611) ;
#14151=AXIS2_PLACEMENT_3D('',#20882,#16614,#16615) ;
#14152=AXIS2_PLACEMENT_3D('',#20884,#16617,#16618) ;
#14153=AXIS2_PLACEMENT_3D('',#20886,#16619,#16620) ;
#14154=AXIS2_PLACEMENT_3D('',#20888,#16622,#16623) ;
#14155=AXIS2_PLACEMENT_3D('',#20892,#16626,#16627) ;
#14156=AXIS2_PLACEMENT_3D('',#20898,#16631,#16632) ;
#14157=AXIS2_PLACEMENT_3D('',#20900,#16634,#16635) ;
#14158=AXIS2_PLACEMENT_3D('',#20902,#16636,#16637) ;
#14159=AXIS2_PLACEMENT_3D('',#20904,#16639,#16640) ;
#14160=AXIS2_PLACEMENT_3D('',#20910,#16644,#16645) ;
#14161=AXIS2_PLACEMENT_3D('',#20914,#16648,#16649) ;
#14162=AXIS2_PLACEMENT_3D('',#20916,#16651,#16652) ;
#14163=AXIS2_PLACEMENT_3D('',#20918,#16653,#16654) ;
#14164=AXIS2_PLACEMENT_3D('',#20920,#16656,#16657) ;
#14165=AXIS2_PLACEMENT_3D('',#20924,#16660,#16661) ;
#14166=AXIS2_PLACEMENT_3D('',#20930,#16665,#16666) ;
#14167=AXIS2_PLACEMENT_3D('',#20932,#16668,#16669) ;
#14168=AXIS2_PLACEMENT_3D('',#20934,#16670,#16671) ;
#14169=AXIS2_PLACEMENT_3D('',#20936,#16673,#16674) ;
#14170=AXIS2_PLACEMENT_3D('',#20942,#16678,#16679) ;
#14171=AXIS2_PLACEMENT_3D('',#20946,#16682,#16683) ;
#14172=AXIS2_PLACEMENT_3D('',#20948,#16685,#16686) ;
#14173=AXIS2_PLACEMENT_3D('',#20950,#16687,#16688) ;
#14174=AXIS2_PLACEMENT_3D('',#20952,#16690,#16691) ;
#14175=AXIS2_PLACEMENT_3D('',#20956,#16694,#16695) ;
#14176=AXIS2_PLACEMENT_3D('',#20962,#16699,#16700) ;
#14177=AXIS2_PLACEMENT_3D('',#20964,#16702,#16703) ;
#14178=AXIS2_PLACEMENT_3D('',#20966,#16704,#16705) ;
#14179=AXIS2_PLACEMENT_3D('',#20968,#16707,#16708) ;
#14180=AXIS2_PLACEMENT_3D('',#20974,#16712,#16713) ;
#14181=AXIS2_PLACEMENT_3D('',#20978,#16716,#16717) ;
#14182=AXIS2_PLACEMENT_3D('',#20980,#16719,#16720) ;
#14183=AXIS2_PLACEMENT_3D('',#20982,#16721,#16722) ;
#14184=AXIS2_PLACEMENT_3D('',#20984,#16724,#16725) ;
#14185=AXIS2_PLACEMENT_3D('',#20988,#16728,#16729) ;
#14186=AXIS2_PLACEMENT_3D('',#20994,#16733,#16734) ;
#14187=AXIS2_PLACEMENT_3D('',#20996,#16736,#16737) ;
#14188=AXIS2_PLACEMENT_3D('',#20998,#16738,#16739) ;
#14189=AXIS2_PLACEMENT_3D('',#21000,#16741,#16742) ;
#14190=AXIS2_PLACEMENT_3D('',#21006,#16746,#16747) ;
#14191=AXIS2_PLACEMENT_3D('',#21010,#16750,#16751) ;
#14192=AXIS2_PLACEMENT_3D('',#21012,#16753,#16754) ;
#14193=AXIS2_PLACEMENT_3D('',#21014,#16755,#16756) ;
#14194=AXIS2_PLACEMENT_3D('',#21016,#16758,#16759) ;
#14195=AXIS2_PLACEMENT_3D('',#21020,#16762,#16763) ;
#14196=AXIS2_PLACEMENT_3D('',#21024,#16766,#16767) ;
#14197=AXIS2_PLACEMENT_3D('',#21026,#16769,#16770) ;
#14198=AXIS2_PLACEMENT_3D('',#21028,#16771,#16772) ;
#14199=AXIS2_PLACEMENT_3D('',#21030,#16774,#16775) ;
#16475=DIRECTION('axis',(0.,0.,1.)) ;
#16476=DIRECTION('refdir',(1.,0.,0.)) ;
#16477=DIRECTION('center_axis',(0.,0.,1.)) ;
#16478=DIRECTION('ref_axis',(1.,0.,0.)) ;
#16479=DIRECTION('',(-1.,0.,0.)) ;
#16480=DIRECTION('',(0.,1.,0.)) ;
#16481=DIRECTION('',(1.,0.,0.)) ;
#16482=DIRECTION('',(0.,-1.,0.)) ;
#16483=DIRECTION('center_axis',(0.,0.,1.)) ;
#16484=DIRECTION('ref_axis',(1.,0.,0.)) ;
#16485=DIRECTION('',(1.,0.,0.)) ;
#16486=DIRECTION('',(0.,1.,0.)) ;
#16487=DIRECTION('',(-1.,0.,0.)) ;
#16488=DIRECTION('',(0.,-1.,0.)) ;
#16489=DIRECTION('center_axis',(-1.,0.,0.)) ;
#16490=DIRECTION('ref_axis',(0.,0.,1.)) ;
#16491=DIRECTION('',(0.,0.,1.)) ;
#16492=DIRECTION('',(0.,0.,-1.)) ;
#16493=DIRECTION('center_axis',(0.,-1.,0.)) ;
#16494=DIRECTION('ref_axis',(-1.,0.,0.)) ;
#16495=DIRECTION('center_axis',(0.,-1.,0.)) ;
#16496=DIRECTION('ref_axis',(1.,0.,0.)) ;
#16497=DIRECTION('center_axis',(0.,1.,0.)) ;
#16498=DIRECTION('ref_axis',(1.,0.,0.)) ;
#16499=DIRECTION('center_axis',(0.,1.,0.)) ;
#16500=DIRECTION('ref_axis',(-1.,0.,1.22464679914735E-16)) ;
#16501=DIRECTION('center_axis',(0.,-1.,0.)) ;
#16502=DIRECTION('ref_axis',(1.,0.,0.)) ;
#16503=DIRECTION('center_axis',(0.5,0.,0.866025403784438)) ;
#16504=DIRECTION('ref_axis',(0.866025403784438,0.,-0.5)) ;
#16505=DIRECTION('',(0.,-1.,0.)) ;
#16506=DIRECTION('',(0.866025403784438,0.,-0.5)) ;
#16507=DIRECTION('',(0.,-1.,0.)) ;
#16508=DIRECTION('',(-0.866025403784438,0.,0.5)) ;
#16509=DIRECTION('center_axis',(0.5,0.,0.866025403784438)) ;
#16510=DIRECTION('ref_axis',(0.866025403784438,0.,-0.5)) ;
#16511=DIRECTION('',(0.,1.,0.)) ;
#16512=DIRECTION('',(0.866025403784438,0.,-0.5)) ;
#16513=DIRECTION('',(0.,1.,0.)) ;
#16514=DIRECTION('',(-0.866025403784438,0.,0.5)) ;
#16515=DIRECTION('center_axis',(-0.866025403784438,0.,0.5)) ;
#16516=DIRECTION('ref_axis',(0.5,0.,0.866025403784438)) ;
#16517=DIRECTION('',(-0.5,0.,-0.866025403784438)) ;
#16518=DIRECTION('',(-0.5,0.,-0.866025403784438)) ;
#16519=DIRECTION('center_axis',(0.,1.,0.)) ;
#16520=DIRECTION('ref_axis',(1.,0.,0.)) ;
#16521=DIRECTION('center_axis',(0.,-1.,0.)) ;
#16522=DIRECTION('ref_axis',(1.,0.,0.)) ;
#16523=DIRECTION('',(0.,1.,0.)) ;
#16524=DIRECTION('center_axis',(0.,1.,0.)) ;
#16525=DIRECTION('ref_axis',(1.,0.,0.)) ;
#16526=DIRECTION('center_axis',(0.,1.,0.)) ;
#16527=DIRECTION('ref_axis',(1.,0.,0.)) ;
#16528=DIRECTION('center_axis',(0.,1.,0.)) ;
#16529=DIRECTION('ref_axis',(1.,0.,0.)) ;
#16530=DIRECTION('',(0.,-1.,0.)) ;
#16531=DIRECTION('center_axis',(0.,-1.,0.)) ;
#16532=DIRECTION('ref_axis',(1.,0.,0.)) ;
#16533=DIRECTION('center_axis',(0.,1.,0.)) ;
#16534=DIRECTION('ref_axis',(1.,0.,0.)) ;
#16535=DIRECTION('',(-0.5,0.,0.866025403784439)) ;
#16536=DIRECTION('',(-0.866025403784439,0.,-0.5)) ;
#16537=DIRECTION('',(0.5,0.,-0.866025403784439)) ;
#16538=DIRECTION('center_axis',(0.,1.,0.)) ;
#16539=DIRECTION('ref_axis',(1.,0.,0.)) ;
#16540=DIRECTION('',(1.83697019872103E-16,0.,1.)) ;
#16541=DIRECTION('',(-1.,0.,1.83697019872103E-16)) ;
#16542=DIRECTION('',(-1.83697019872103E-16,0.,-1.)) ;
#16543=DIRECTION('center_axis',(0.,1.,0.)) ;
#16544=DIRECTION('ref_axis',(1.,0.,0.)) ;
#16545=DIRECTION('',(0.5,0.,0.866025403784438)) ;
#16546=DIRECTION('',(-0.866025403784438,0.,0.5)) ;
#16547=DIRECTION('',(-0.5,0.,-0.866025403784438)) ;
#16548=DIRECTION('center_axis',(0.,1.,0.)) ;
#16549=DIRECTION('ref_axis',(1.,0.,0.)) ;
#16550=DIRECTION('',(0.866025403784439,0.,0.5)) ;
#16551=DIRECTION('',(-0.5,0.,0.866025403784439)) ;
#16552=DIRECTION('',(-0.866025403784439,0.,-0.5)) ;
#16553=DIRECTION('center_axis',(0.,1.,0.)) ;
#16554=DIRECTION('ref_axis',(1.,0.,0.)) ;
#16555=DIRECTION('',(1.,0.,-1.22464679914735E-16)) ;
#16556=DIRECTION('',(1.22464679914735E-16,0.,1.)) ;
#16557=DIRECTION('',(-1.,0.,1.22464679914735E-16)) ;
#16558=DIRECTION('center_axis',(0.,1.,0.)) ;
#16559=DIRECTION('ref_axis',(1.,0.,0.)) ;
#16560=DIRECTION('',(0.866025403784439,0.,-0.5)) ;
#16561=DIRECTION('',(0.5,0.,0.866025403784439)) ;
#16562=DIRECTION('',(-0.866025403784439,0.,0.5)) ;
#16563=DIRECTION('center_axis',(0.,1.,0.)) ;
#16564=DIRECTION('ref_axis',(1.,0.,0.)) ;
#16565=DIRECTION('',(0.5,0.,-0.866025403784439)) ;
#16566=DIRECTION('',(0.866025403784439,0.,0.5)) ;
#16567=DIRECTION('',(-0.5,0.,0.866025403784439)) ;
#16568=DIRECTION('center_axis',(0.,1.,0.)) ;
#16569=DIRECTION('ref_axis',(1.,0.,0.)) ;
#16570=DIRECTION('',(-6.12323399573677E-17,0.,-1.)) ;
#16571=DIRECTION('',(1.,0.,-6.12323399573677E-17)) ;
#16572=DIRECTION('',(6.12323399573677E-17,0.,1.)) ;
#16573=DIRECTION('center_axis',(0.,1.,0.)) ;
#16574=DIRECTION('ref_axis',(1.,0.,0.)) ;
#16575=DIRECTION('',(-0.5,0.,-0.866025403784439)) ;
#16576=DIRECTION('',(0.866025403784439,0.,-0.5)) ;
#16577=DIRECTION('',(0.5,0.,0.866025403784439)) ;
#16578=DIRECTION('center_axis',(0.,1.,0.)) ;
#16579=DIRECTION('ref_axis',(1.,0.,0.)) ;
#16580=DIRECTION('',(-0.866025403784439,0.,-0.5)) ;
#16581=DIRECTION('',(0.5,0.,-0.866025403784439)) ;
#16582=DIRECTION('',(0.866025403784439,0.,0.5)) ;
#16583=DIRECTION('center_axis',(0.,1.,0.)) ;
#16584=DIRECTION('ref_axis',(1.,0.,0.)) ;
#16585=DIRECTION('',(-1.,0.,0.)) ;
#16586=DIRECTION('',(0.,0.,-1.)) ;
#16587=DIRECTION('',(1.,0.,0.)) ;
#16588=DIRECTION('center_axis',(0.866025403784439,0.,0.5)) ;
#16589=DIRECTION('ref_axis',(0.5,0.,-0.866025403784439)) ;
#16590=DIRECTION('',(0.5,0.,-0.866025403784439)) ;
#16591=DIRECTION('',(0.,1.,0.)) ;
#16592=DIRECTION('center_axis',(0.866025403784439,0.,0.5)) ;
#16593=DIRECTION('ref_axis',(0.5,0.,-0.866025403784439)) ;
#16594=DIRECTION('',(0.,-1.,0.)) ;
#16595=DIRECTION('',(0.,-1.,0.)) ;
#16596=DIRECTION('',(-0.5,0.,0.866025403784439)) ;
#16597=DIRECTION('center_axis',(-0.5,0.,0.866025403784439)) ;
#16598=DIRECTION('ref_axis',(0.866025403784439,0.,0.5)) ;
#16599=DIRECTION('',(-0.866025403784439,0.,-0.5)) ;
#16600=DIRECTION('center_axis',(0.,1.,0.)) ;
#16601=DIRECTION('ref_axis',(1.,0.,0.)) ;
#16602=DIRECTION('center_axis',(0.,-1.,0.)) ;
#16603=DIRECTION('ref_axis',(1.,0.,0.)) ;
#16604=DIRECTION('',(0.,1.,0.)) ;
#16605=DIRECTION('center_axis',(1.,0.,-1.83697019872103E-16)) ;
#16606=DIRECTION('ref_axis',(-1.83697019872103E-16,0.,-1.)) ;
#16607=DIRECTION('',(0.,-1.,0.)) ;
#16608=DIRECTION('',(0.,-1.,0.)) ;
#16609=DIRECTION('',(1.83697019872103E-16,0.,1.)) ;
#16610=DIRECTION('center_axis',(1.,0.,-1.83697019872103E-16)) ;
#16611=DIRECTION('ref_axis',(-1.83697019872103E-16,0.,-1.)) ;
#16612=DIRECTION('',(-1.83697019872103E-16,0.,-1.)) ;
#16613=DIRECTION('',(0.,1.,0.)) ;
#16614=DIRECTION('center_axis',(1.83697019872103E-16,0.,1.)) ;
#16615=DIRECTION('ref_axis',(1.,0.,-1.83697019872103E-16)) ;
#16616=DIRECTION('',(-1.,0.,1.83697019872103E-16)) ;
#16617=DIRECTION('center_axis',(0.,1.,0.)) ;
#16618=DIRECTION('ref_axis',(1.,0.,0.)) ;
#16619=DIRECTION('center_axis',(0.,-1.,0.)) ;
#16620=DIRECTION('ref_axis',(1.,0.,0.)) ;
#16621=DIRECTION('',(0.,1.,0.)) ;
#16622=DIRECTION('center_axis',(0.866025403784438,0.,-0.5)) ;
#16623=DIRECTION('ref_axis',(-0.5,0.,-0.866025403784438)) ;
#16624=DIRECTION('',(-0.5,0.,-0.866025403784438)) ;
#16625=DIRECTION('',(0.,1.,0.)) ;
#16626=DIRECTION('center_axis',(0.866025403784438,0.,-0.5)) ;
#16627=DIRECTION('ref_axis',(-0.5,0.,-0.866025403784438)) ;
#16628=DIRECTION('',(0.,-1.,0.)) ;
#16629=DIRECTION('',(0.,-1.,0.)) ;
#16630=DIRECTION('',(0.5,0.,0.866025403784438)) ;
#16631=DIRECTION('center_axis',(0.5,0.,0.866025403784438)) ;
#16632=DIRECTION('ref_axis',(0.866025403784438,0.,-0.5)) ;
#16633=DIRECTION('',(-0.866025403784438,0.,0.5)) ;
#16634=DIRECTION('center_axis',(0.,1.,0.)) ;
#16635=DIRECTION('ref_axis',(1.,0.,0.)) ;
#16636=DIRECTION('center_axis',(0.,-1.,0.)) ;
#16637=DIRECTION('ref_axis',(1.,0.,0.)) ;
#16638=DIRECTION('',(0.,1.,0.)) ;
#16639=DIRECTION('center_axis',(0.5,0.,-0.866025403784439)) ;
#16640=DIRECTION('ref_axis',(-0.866025403784439,0.,-0.5)) ;
#16641=DIRECTION('',(0.,-1.,0.)) ;
#16642=DIRECTION('',(0.,-1.,0.)) ;
#16643=DIRECTION('',(0.866025403784439,0.,0.5)) ;
#16644=DIRECTION('center_axis',(0.5,0.,-0.866025403784439)) ;
#16645=DIRECTION('ref_axis',(-0.866025403784439,0.,-0.5)) ;
#16646=DIRECTION('',(-0.866025403784439,0.,-0.5)) ;
#16647=DIRECTION('',(0.,1.,0.)) ;
#16648=DIRECTION('center_axis',(0.866025403784439,0.,0.5)) ;
#16649=DIRECTION('ref_axis',(0.5,0.,-0.866025403784439)) ;
#16650=DIRECTION('',(-0.5,0.,0.866025403784439)) ;
#16651=DIRECTION('center_axis',(0.,1.,0.)) ;
#16652=DIRECTION('ref_axis',(1.,0.,0.)) ;
#16653=DIRECTION('center_axis',(0.,-1.,0.)) ;
#16654=DIRECTION('ref_axis',(1.,0.,0.)) ;
#16655=DIRECTION('',(0.,1.,0.)) ;
#16656=DIRECTION('center_axis',(-1.22464679914735E-16,0.,-1.)) ;
#16657=DIRECTION('ref_axis',(-1.,0.,1.22464679914735E-16)) ;
#16658=DIRECTION('',(-1.,0.,1.22464679914735E-16)) ;
#16659=DIRECTION('',(0.,1.,0.)) ;
#16660=DIRECTION('center_axis',(-1.22464679914735E-16,0.,-1.)) ;
#16661=DIRECTION('ref_axis',(-1.,0.,1.22464679914735E-16)) ;
#16662=DIRECTION('',(0.,-1.,0.)) ;
#16663=DIRECTION('',(0.,-1.,0.)) ;
#16664=DIRECTION('',(1.,0.,-1.22464679914735E-16)) ;
#16665=DIRECTION('center_axis',(1.,0.,-1.22464679914735E-16)) ;
#16666=DIRECTION('ref_axis',(-1.22464679914735E-16,0.,-1.)) ;
#16667=DIRECTION('',(1.22464679914735E-16,0.,1.)) ;
#16668=DIRECTION('center_axis',(0.,1.,0.)) ;
#16669=DIRECTION('ref_axis',(1.,0.,0.)) ;
#16670=DIRECTION('center_axis',(0.,-1.,0.)) ;
#16671=DIRECTION('ref_axis',(1.,0.,0.)) ;
#16672=DIRECTION('',(0.,1.,0.)) ;
#16673=DIRECTION('center_axis',(-0.5,0.,-0.866025403784439)) ;
#16674=DIRECTION('ref_axis',(-0.866025403784439,0.,0.5)) ;
#16675=DIRECTION('',(0.,-1.,0.)) ;
#16676=DIRECTION('',(0.,-1.,0.)) ;
#16677=DIRECTION('',(0.866025403784439,0.,-0.5)) ;
#16678=DIRECTION('center_axis',(-0.5,0.,-0.866025403784439)) ;
#16679=DIRECTION('ref_axis',(-0.866025403784439,0.,0.5)) ;
#16680=DIRECTION('',(-0.866025403784439,0.,0.5)) ;
#16681=DIRECTION('',(0.,1.,0.)) ;
#16682=DIRECTION('center_axis',(0.866025403784439,0.,-0.5)) ;
#16683=DIRECTION('ref_axis',(-0.5,0.,-0.866025403784439)) ;
#16684=DIRECTION('',(0.5,0.,0.866025403784439)) ;
#16685=DIRECTION('center_axis',(0.,1.,0.)) ;
#16686=DIRECTION('ref_axis',(1.,0.,0.)) ;
#16687=DIRECTION('center_axis',(0.,-1.,0.)) ;
#16688=DIRECTION('ref_axis',(1.,0.,0.)) ;
#16689=DIRECTION('',(0.,1.,0.)) ;
#16690=DIRECTION('center_axis',(-0.866025403784439,0.,-0.5)) ;
#16691=DIRECTION('ref_axis',(-0.5,0.,0.866025403784439)) ;
#16692=DIRECTION('',(-0.5,0.,0.866025403784439)) ;
#16693=DIRECTION('',(0.,1.,0.)) ;
#16694=DIRECTION('center_axis',(-0.866025403784439,0.,-0.5)) ;
#16695=DIRECTION('ref_axis',(-0.5,0.,0.866025403784439)) ;
#16696=DIRECTION('',(0.,-1.,0.)) ;
#16697=DIRECTION('',(0.,-1.,0.)) ;
#16698=DIRECTION('',(0.5,0.,-0.866025403784439)) ;
#16699=DIRECTION('center_axis',(0.5,0.,-0.866025403784439)) ;
#16700=DIRECTION('ref_axis',(-0.866025403784439,0.,-0.5)) ;
#16701=DIRECTION('',(0.866025403784439,0.,0.5)) ;
#16702=DIRECTION('center_axis',(0.,1.,0.)) ;
#16703=DIRECTION('ref_axis',(1.,0.,0.)) ;
#16704=DIRECTION('center_axis',(0.,-1.,0.)) ;
#16705=DIRECTION('ref_axis',(1.,0.,0.)) ;
#16706=DIRECTION('',(0.,1.,0.)) ;
#16707=DIRECTION('center_axis',(-1.,0.,6.12323399573677E-17)) ;
#16708=DIRECTION('ref_axis',(6.12323399573677E-17,0.,1.)) ;
#16709=DIRECTION('',(0.,-1.,0.)) ;
#16710=DIRECTION('',(0.,-1.,0.)) ;
#16711=DIRECTION('',(-6.12323399573677E-17,0.,-1.)) ;
#16712=DIRECTION('center_axis',(-1.,0.,6.12323399573677E-17)) ;
#16713=DIRECTION('ref_axis',(6.12323399573677E-17,0.,1.)) ;
#16714=DIRECTION('',(6.12323399573677E-17,0.,1.)) ;
#16715=DIRECTION('',(0.,1.,0.)) ;
#16716=DIRECTION('center_axis',(-6.12323399573677E-17,0.,-1.)) ;
#16717=DIRECTION('ref_axis',(-1.,0.,6.12323399573677E-17)) ;
#16718=DIRECTION('',(1.,0.,-6.12323399573677E-17)) ;
#16719=DIRECTION('center_axis',(0.,1.,0.)) ;
#16720=DIRECTION('ref_axis',(1.,0.,0.)) ;
#16721=DIRECTION('center_axis',(0.,-1.,0.)) ;
#16722=DIRECTION('ref_axis',(1.,0.,0.)) ;
#16723=DIRECTION('',(0.,1.,0.)) ;
#16724=DIRECTION('center_axis',(-0.866025403784439,0.,0.5)) ;
#16725=DIRECTION('ref_axis',(0.5,0.,0.866025403784439)) ;
#16726=DIRECTION('',(0.5,0.,0.866025403784439)) ;
#16727=DIRECTION('',(0.,1.,0.)) ;
#16728=DIRECTION('center_axis',(-0.866025403784439,0.,0.5)) ;
#16729=DIRECTION('ref_axis',(0.5,0.,0.866025403784439)) ;
#16730=DIRECTION('',(0.,-1.,0.)) ;
#16731=DIRECTION('',(0.,-1.,0.)) ;
#16732=DIRECTION('',(-0.5,0.,-0.866025403784439)) ;
#16733=DIRECTION('center_axis',(-0.5,0.,-0.866025403784439)) ;
#16734=DIRECTION('ref_axis',(-0.866025403784439,0.,0.5)) ;
#16735=DIRECTION('',(0.866025403784439,0.,-0.5)) ;
#16736=DIRECTION('center_axis',(0.,1.,0.)) ;
#16737=DIRECTION('ref_axis',(1.,0.,0.)) ;
#16738=DIRECTION('center_axis',(0.,-1.,0.)) ;
#16739=DIRECTION('ref_axis',(1.,0.,0.)) ;
#16740=DIRECTION('',(0.,1.,0.)) ;
#16741=DIRECTION('center_axis',(-0.5,0.,0.866025403784439)) ;
#16742=DIRECTION('ref_axis',(0.866025403784439,0.,0.5)) ;
#16743=DIRECTION('',(0.,-1.,0.)) ;
#16744=DIRECTION('',(0.,-1.,0.)) ;
#16745=DIRECTION('',(-0.866025403784439,0.,-0.5)) ;
#16746=DIRECTION('center_axis',(-0.5,0.,0.866025403784439)) ;
#16747=DIRECTION('ref_axis',(0.866025403784439,0.,0.5)) ;
#16748=DIRECTION('',(0.866025403784439,0.,0.5)) ;
#16749=DIRECTION('',(0.,1.,0.)) ;
#16750=DIRECTION('center_axis',(-0.866025403784439,0.,-0.5)) ;
#16751=DIRECTION('ref_axis',(-0.5,0.,0.866025403784439)) ;
#16752=DIRECTION('',(0.5,0.,-0.866025403784439)) ;
#16753=DIRECTION('center_axis',(0.,1.,0.)) ;
#16754=DIRECTION('ref_axis',(1.,0.,0.)) ;
#16755=DIRECTION('center_axis',(0.,-1.,0.)) ;
#16756=DIRECTION('ref_axis',(1.,0.,0.)) ;
#16757=DIRECTION('',(0.,1.,0.)) ;
#16758=DIRECTION('center_axis',(0.,0.,1.)) ;
#16759=DIRECTION('ref_axis',(1.,0.,0.)) ;
#16760=DIRECTION('',(1.,0.,0.)) ;
#16761=DIRECTION('',(0.,1.,0.)) ;
#16762=DIRECTION('center_axis',(0.,0.,1.)) ;
#16763=DIRECTION('ref_axis',(1.,0.,0.)) ;
#16764=DIRECTION('',(0.,-1.,0.)) ;
#16765=DIRECTION('',(-1.,0.,0.)) ;
#16766=DIRECTION('center_axis',(-1.,0.,0.)) ;
#16767=DIRECTION('ref_axis',(0.,0.,1.)) ;
#16768=DIRECTION('',(0.,0.,-1.)) ;
#16769=DIRECTION('center_axis',(0.,1.,0.)) ;
#16770=DIRECTION('ref_axis',(1.,0.,0.)) ;
#16771=DIRECTION('center_axis',(0.,1.,0.)) ;
#16772=DIRECTION('ref_axis',(1.,0.,0.)) ;
#16773=DIRECTION('',(0.,-1.,0.)) ;
#16774=DIRECTION('center_axis',(0.,-1.,0.)) ;
#16775=DIRECTION('ref_axis',(-1.,0.,0.)) ;
#20709=CARTESIAN_POINT('',(0.,0.,0.)) ;
#20710=CARTESIAN_POINT('Origin',(0.83,-6.25,0.252)) ;
#20711=CARTESIAN_POINT('',(1.01,-5.7,0.252)) ;
#20712=CARTESIAN_POINT('',(0.706396489232499,-5.7,0.252)) ;
#20713=CARTESIAN_POINT('',(0.415,-5.7,0.252)) ;
#20714=CARTESIAN_POINT('',(1.01,-6.8,0.252)) ;
#20715=CARTESIAN_POINT('',(1.01,-6.25,0.252)) ;
#20716=CARTESIAN_POINT('',(0.706396489232499,-6.8,0.252)) ;
#20717=CARTESIAN_POINT('',(0.415,-6.8,0.252)) ;
#20718=CARTESIAN_POINT('',(0.706396489232499,-6.25,0.252)) ;
#20719=CARTESIAN_POINT('Origin',(0.83,-6.25,-0.252)) ;
#20720=CARTESIAN_POINT('',(0.706396489232499,-5.7,-0.252)) ;
#20721=CARTESIAN_POINT('',(1.01,-5.7,-0.252)) ;
#20722=CARTESIAN_POINT('',(0.415,-5.7,-0.252)) ;
#20723=CARTESIAN_POINT('',(0.706396489232499,-6.8,-0.252)) ;
#20724=CARTESIAN_POINT('',(0.706396489232499,-6.25,-0.252)) ;
#20725=CARTESIAN_POINT('',(1.01,-6.8,-0.252)) ;
#20726=CARTESIAN_POINT('',(0.415,-6.8,-0.252)) ;
#20727=CARTESIAN_POINT('',(1.01,-6.25,-0.252)) ;
#20728=CARTESIAN_POINT('Origin',(1.01,-6.25,0.)) ;
#20729=CARTESIAN_POINT('',(1.01,-5.7,0.)) ;
#20730=CARTESIAN_POINT('',(1.01,-6.8,0.)) ;
#20731=CARTESIAN_POINT('Origin',(0.,-6.8,0.)) ;
#20732=CARTESIAN_POINT('',(-1.4,-6.8,1.71450551880629E-16)) ;
#20733=CARTESIAN_POINT('Origin',(0.,-6.8,0.)) ;
#20734=CARTESIAN_POINT('Origin',(0.,-6.8,0.)) ;
#20735=CARTESIAN_POINT('Origin',(0.,-6.25,0.)) ;
#20736=CARTESIAN_POINT('Origin',(0.,-5.7,0.)) ;
#20737=CARTESIAN_POINT('Origin',(2.21326859021798,-6.05,-1.56650635094611)) ;
#20738=CARTESIAN_POINT('',(2.02921099245176,-5.7,-1.46024064732939)) ;
#20739=CARTESIAN_POINT('',(2.02921099245176,-6.4,-1.46024064732939)) ;
#20740=CARTESIAN_POINT('',(2.02921099245176,-6.05,-1.46024064732939)) ;
#20741=CARTESIAN_POINT('',(2.47307621135332,-5.7,-1.71650635094611)) ;
#20742=CARTESIAN_POINT('',(2.21326859021798,-5.7,-1.56650635094611)) ;
#20743=CARTESIAN_POINT('',(2.47307621135332,-6.4,-1.71650635094611)) ;
#20744=CARTESIAN_POINT('',(2.47307621135332,-6.05,-1.71650635094611)) ;
#20745=CARTESIAN_POINT('',(2.21326859021798,-6.4,-1.56650635094611)) ;
#20746=CARTESIAN_POINT('Origin',(2.46326859021798,-6.05,-1.13349364905389)) ;
#20747=CARTESIAN_POINT('',(2.27921099245176,-6.4,-1.02722794543717)) ;
#20748=CARTESIAN_POINT('',(2.27921099245176,-5.7,-1.02722794543717)) ;
#20749=CARTESIAN_POINT('',(2.27921099245176,-6.05,-1.02722794543717)) ;
#20750=CARTESIAN_POINT('',(2.72307621135332,-6.4,-1.28349364905389)) ;
#20751=CARTESIAN_POINT('',(2.46326859021798,-6.4,-1.13349364905389)) ;
#20752=CARTESIAN_POINT('',(2.72307621135332,-5.7,-1.28349364905389)) ;
#20753=CARTESIAN_POINT('',(2.72307621135332,-6.05,-1.28349364905389)) ;
#20754=CARTESIAN_POINT('',(2.46326859021798,-5.7,-1.13349364905389)) ;
#20755=CARTESIAN_POINT('Origin',(2.59807621135332,-6.05,-1.5)) ;
#20756=CARTESIAN_POINT('',(2.59807621135332,-6.4,-1.5)) ;
#20757=CARTESIAN_POINT('',(2.59807621135332,-5.7,-1.5)) ;
#20758=CARTESIAN_POINT('Origin',(0.,-6.05,0.)) ;
#20759=CARTESIAN_POINT('',(1.46024064732938,-6.4,-2.02921099245176)) ;
#20760=CARTESIAN_POINT('Origin',(0.,-6.4,0.)) ;
#20761=CARTESIAN_POINT('',(1.46024064732938,-5.7,-2.02921099245176)) ;
#20762=CARTESIAN_POINT('',(1.46024064732938,-6.05,-2.02921099245176)) ;
#20763=CARTESIAN_POINT('Origin',(0.,-5.7,0.)) ;
#20764=CARTESIAN_POINT('Origin',(0.,-6.05,0.)) ;
#20765=CARTESIAN_POINT('',(2.48746859276655,-5.7,-0.25)) ;
#20766=CARTESIAN_POINT('Origin',(0.,-5.7,0.)) ;
#20767=CARTESIAN_POINT('',(2.48746859276655,-6.4,-0.25)) ;
#20768=CARTESIAN_POINT('',(2.48746859276655,-6.05,-0.25)) ;
#20769=CARTESIAN_POINT('Origin',(0.,-6.4,0.)) ;
#20770=CARTESIAN_POINT('Origin',(0.,-5.7,0.)) ;
#20771=CARTESIAN_POINT('',(1.71650635094611,-5.7,-2.47307621135332)) ;
#20772=CARTESIAN_POINT('',(1.56650635094611,-5.7,-2.21326859021798)) ;
#20773=CARTESIAN_POINT('',(1.28349364905389,-5.7,-2.72307621135332)) ;
#20774=CARTESIAN_POINT('',(1.5,-5.7,-2.59807621135332)) ;
#20775=CARTESIAN_POINT('',(1.02722794543717,-5.7,-2.27921099245176)) ;
#20776=CARTESIAN_POINT('',(1.13349364905389,-5.7,-2.46326859021798)) ;
#20777=CARTESIAN_POINT('',(0.25,-5.7,-2.48746859276655)) ;
#20778=CARTESIAN_POINT('Origin',(0.,-5.7,0.)) ;
#20779=CARTESIAN_POINT('',(0.249999999999999,-5.7,-3.)) ;
#20780=CARTESIAN_POINT('',(0.25,-5.7,-2.7)) ;
#20781=CARTESIAN_POINT('',(-0.250000000000001,-5.7,-3.)) ;
#20782=CARTESIAN_POINT('',(-5.51091059616309E-16,-5.7,-3.)) ;
#20783=CARTESIAN_POINT('',(-0.25,-5.7,-2.48746859276655)) ;
#20784=CARTESIAN_POINT('',(-0.25,-5.7,-2.7)) ;
#20785=CARTESIAN_POINT('',(-1.02722794543717,-5.7,-2.27921099245176)) ;
#20786=CARTESIAN_POINT('Origin',(0.,-5.7,0.)) ;
#20787=CARTESIAN_POINT('',(-1.28349364905389,-5.7,-2.72307621135332)) ;
#20788=CARTESIAN_POINT('',(-1.13349364905389,-5.7,-2.46326859021798)) ;
#20789=CARTESIAN_POINT('',(-1.71650635094611,-5.7,-2.47307621135332)) ;
#20790=CARTESIAN_POINT('',(-1.5,-5.7,-2.59807621135332)) ;
#20791=CARTESIAN_POINT('',(-1.46024064732939,-5.7,-2.02921099245176)) ;
#20792=CARTESIAN_POINT('',(-1.56650635094611,-5.7,-2.21326859021798)) ;
#20793=CARTESIAN_POINT('',(-2.02921099245176,-5.7,-1.46024064732938)) ;
#20794=CARTESIAN_POINT('Origin',(0.,-5.7,0.)) ;
#20795=CARTESIAN_POINT('',(-2.47307621135332,-5.7,-1.71650635094611)) ;
#20796=CARTESIAN_POINT('',(-2.21326859021798,-5.7,-1.56650635094611)) ;
#20797=CARTESIAN_POINT('',(-2.72307621135332,-5.7,-1.28349364905389)) ;
#20798=CARTESIAN_POINT('',(-2.59807621135332,-5.7,-1.5)) ;
#20799=CARTESIAN_POINT('',(-2.27921099245176,-5.7,-1.02722794543717)) ;
#20800=CARTESIAN_POINT('',(-2.46326859021798,-5.7,-1.13349364905389)) ;
#20801=CARTESIAN_POINT('',(-2.48746859276655,-5.7,-0.25)) ;
#20802=CARTESIAN_POINT('Origin',(0.,-5.7,0.)) ;
#20803=CARTESIAN_POINT('',(-3.,-5.7,-0.25)) ;
#20804=CARTESIAN_POINT('',(-2.7,-5.7,-0.25)) ;
#20805=CARTESIAN_POINT('',(-3.,-5.7,0.25)) ;
#20806=CARTESIAN_POINT('',(-3.,-5.7,3.67394039744206E-16)) ;
#20807=CARTESIAN_POINT('',(-2.48746859276655,-5.7,0.25)) ;
#20808=CARTESIAN_POINT('',(-2.7,-5.7,0.25)) ;
#20809=CARTESIAN_POINT('',(-2.27921099245176,-5.7,1.02722794543716)) ;
#20810=CARTESIAN_POINT('Origin',(0.,-5.7,0.)) ;
#20811=CARTESIAN_POINT('',(-2.72307621135332,-5.7,1.28349364905389)) ;
#20812=CARTESIAN_POINT('',(-2.46326859021798,-5.7,1.13349364905389)) ;
#20813=CARTESIAN_POINT('',(-2.47307621135332,-5.7,1.71650635094611)) ;
#20814=CARTESIAN_POINT('',(-2.59807621135332,-5.7,1.5)) ;
#20815=CARTESIAN_POINT('',(-2.02921099245176,-5.7,1.46024064732938)) ;
#20816=CARTESIAN_POINT('',(-2.21326859021798,-5.7,1.56650635094611)) ;
#20817=CARTESIAN_POINT('',(-1.46024064732938,-5.7,2.02921099245176)) ;
#20818=CARTESIAN_POINT('Origin',(0.,-5.7,0.)) ;
#20819=CARTESIAN_POINT('',(-1.71650635094611,-5.7,2.47307621135332)) ;
#20820=CARTESIAN_POINT('',(-1.56650635094611,-5.7,2.21326859021798)) ;
#20821=CARTESIAN_POINT('',(-1.28349364905389,-5.7,2.72307621135332)) ;
#20822=CARTESIAN_POINT('',(-1.5,-5.7,2.59807621135332)) ;
#20823=CARTESIAN_POINT('',(-1.02722794543716,-5.7,2.27921099245176)) ;
#20824=CARTESIAN_POINT('',(-1.13349364905389,-5.7,2.46326859021798)) ;
#20825=CARTESIAN_POINT('',(-0.25,-5.7,2.48746859276655)) ;
#20826=CARTESIAN_POINT('Origin',(0.,-5.7,0.)) ;
#20827=CARTESIAN_POINT('',(-0.25,-5.7,3.)) ;
#20828=CARTESIAN_POINT('',(-0.25,-5.7,2.7)) ;
#20829=CARTESIAN_POINT('',(0.25,-5.7,3.)) ;
#20830=CARTESIAN_POINT('',(1.83697019872103E-16,-5.7,3.)) ;
#20831=CARTESIAN_POINT('',(0.25,-5.7,2.48746859276655)) ;
#20832=CARTESIAN_POINT('',(0.25,-5.7,2.7)) ;
#20833=CARTESIAN_POINT('',(1.02722794543717,-5.7,2.27921099245176)) ;
#20834=CARTESIAN_POINT('Origin',(0.,-5.7,0.)) ;
#20835=CARTESIAN_POINT('',(1.28349364905389,-5.7,2.72307621135332)) ;
#20836=CARTESIAN_POINT('',(1.13349364905389,-5.7,2.46326859021798)) ;
#20837=CARTESIAN_POINT('',(1.71650635094611,-5.7,2.47307621135332)) ;
#20838=CARTESIAN_POINT('',(1.5,-5.7,2.59807621135332)) ;
#20839=CARTESIAN_POINT('',(1.46024064732938,-5.7,2.02921099245176)) ;
#20840=CARTESIAN_POINT('',(1.56650635094611,-5.7,2.21326859021798)) ;
#20841=CARTESIAN_POINT('',(2.02921099245176,-5.7,1.46024064732938)) ;
#20842=CARTESIAN_POINT('Origin',(0.,-5.7,0.)) ;
#20843=CARTESIAN_POINT('',(2.47307621135332,-5.7,1.71650635094611)) ;
#20844=CARTESIAN_POINT('',(2.21326859021798,-5.7,1.56650635094611)) ;
#20845=CARTESIAN_POINT('',(2.72307621135332,-5.7,1.28349364905389)) ;
#20846=CARTESIAN_POINT('',(2.59807621135332,-5.7,1.5)) ;
#20847=CARTESIAN_POINT('',(2.27921099245176,-5.7,1.02722794543716)) ;
#20848=CARTESIAN_POINT('',(2.46326859021798,-5.7,1.13349364905389)) ;
#20849=CARTESIAN_POINT('',(2.48746859276655,-5.7,0.25)) ;
#20850=CARTESIAN_POINT('Origin',(0.,-5.7,0.)) ;
#20851=CARTESIAN_POINT('',(3.,-5.7,0.25)) ;
#20852=CARTESIAN_POINT('',(2.7,-5.7,0.25)) ;
#20853=CARTESIAN_POINT('',(3.,-5.7,-0.25)) ;
#20854=CARTESIAN_POINT('',(3.,-5.7,0.)) ;
#20855=CARTESIAN_POINT('',(2.7,-5.7,-0.25)) ;
#20856=CARTESIAN_POINT('Origin',(1.56650635094611,-6.05,-2.21326859021798)) ;
#20857=CARTESIAN_POINT('',(1.71650635094611,-6.4,-2.47307621135332)) ;
#20858=CARTESIAN_POINT('',(1.56650635094611,-6.4,-2.21326859021798)) ;
#20859=CARTESIAN_POINT('',(1.71650635094611,-6.05,-2.47307621135332)) ;
#20860=CARTESIAN_POINT('Origin',(1.13349364905389,-6.05,-2.46326859021798)) ;
#20861=CARTESIAN_POINT('',(1.02722794543717,-6.4,-2.27921099245176)) ;
#20862=CARTESIAN_POINT('',(1.02722794543717,-6.05,-2.27921099245176)) ;
#20863=CARTESIAN_POINT('',(1.28349364905389,-6.4,-2.72307621135332)) ;
#20864=CARTESIAN_POINT('',(1.28349364905389,-6.05,-2.72307621135332)) ;
#20865=CARTESIAN_POINT('',(1.13349364905389,-6.4,-2.46326859021798)) ;
#20866=CARTESIAN_POINT('Origin',(1.5,-6.05,-2.59807621135332)) ;
#20867=CARTESIAN_POINT('',(1.5,-6.4,-2.59807621135332)) ;
#20868=CARTESIAN_POINT('Origin',(0.,-6.05,0.)) ;
#20869=CARTESIAN_POINT('',(0.25,-6.4,-2.48746859276655)) ;
#20870=CARTESIAN_POINT('Origin',(0.,-6.4,0.)) ;
#20871=CARTESIAN_POINT('',(0.25,-6.05,-2.48746859276655)) ;
#20872=CARTESIAN_POINT('Origin',(-0.25,-6.05,-2.7)) ;
#20873=CARTESIAN_POINT('',(-0.25,-6.4,-2.48746859276655)) ;
#20874=CARTESIAN_POINT('',(-0.25,-6.05,-2.48746859276655)) ;
#20875=CARTESIAN_POINT('',(-0.250000000000001,-6.4,-3.)) ;
#20876=CARTESIAN_POINT('',(-0.250000000000001,-6.05,-3.)) ;
#20877=CARTESIAN_POINT('',(-0.25,-6.4,-2.7)) ;
#20878=CARTESIAN_POINT('Origin',(0.25,-6.05,-2.7)) ;
#20879=CARTESIAN_POINT('',(0.249999999999999,-6.4,-3.)) ;
#20880=CARTESIAN_POINT('',(0.25,-6.4,-2.7)) ;
#20881=CARTESIAN_POINT('',(0.249999999999999,-6.05,-3.)) ;
#20882=CARTESIAN_POINT('Origin',(-5.51091059616309E-16,-6.05,-3.)) ;
#20883=CARTESIAN_POINT('',(-5.51091059616309E-16,-6.4,-3.)) ;
#20884=CARTESIAN_POINT('Origin',(0.,-6.05,0.)) ;
#20885=CARTESIAN_POINT('',(-1.02722794543717,-6.4,-2.27921099245176)) ;
#20886=CARTESIAN_POINT('Origin',(0.,-6.4,0.)) ;
#20887=CARTESIAN_POINT('',(-1.02722794543717,-6.05,-2.27921099245176)) ;
#20888=CARTESIAN_POINT('Origin',(-1.13349364905389,-6.05,-2.46326859021798)) ;
#20889=CARTESIAN_POINT('',(-1.28349364905389,-6.4,-2.72307621135332)) ;
#20890=CARTESIAN_POINT('',(-1.13349364905389,-6.4,-2.46326859021798)) ;
#20891=CARTESIAN_POINT('',(-1.28349364905389,-6.05,-2.72307621135332)) ;
#20892=CARTESIAN_POINT('Origin',(-1.56650635094611,-6.05,-2.21326859021798)) ;
#20893=CARTESIAN_POINT('',(-1.46024064732939,-6.4,-2.02921099245176)) ;
#20894=CARTESIAN_POINT('',(-1.46024064732939,-6.05,-2.02921099245176)) ;
#20895=CARTESIAN_POINT('',(-1.71650635094611,-6.4,-2.47307621135332)) ;
#20896=CARTESIAN_POINT('',(-1.71650635094611,-6.05,-2.47307621135332)) ;
#20897=CARTESIAN_POINT('',(-1.56650635094611,-6.4,-2.21326859021798)) ;
#20898=CARTESIAN_POINT('Origin',(-1.5,-6.05,-2.59807621135332)) ;
#20899=CARTESIAN_POINT('',(-1.5,-6.4,-2.59807621135332)) ;
#20900=CARTESIAN_POINT('Origin',(0.,-6.05,0.)) ;
#20901=CARTESIAN_POINT('',(-2.02921099245176,-6.4,-1.46024064732938)) ;
#20902=CARTESIAN_POINT('Origin',(0.,-6.4,0.)) ;
#20903=CARTESIAN_POINT('',(-2.02921099245176,-6.05,-1.46024064732938)) ;
#20904=CARTESIAN_POINT('Origin',(-2.46326859021798,-6.05,-1.13349364905389)) ;
#20905=CARTESIAN_POINT('',(-2.27921099245176,-6.4,-1.02722794543717)) ;
#20906=CARTESIAN_POINT('',(-2.27921099245176,-6.05,-1.02722794543717)) ;
#20907=CARTESIAN_POINT('',(-2.72307621135332,-6.4,-1.28349364905389)) ;
#20908=CARTESIAN_POINT('',(-2.72307621135332,-6.05,-1.28349364905389)) ;
#20909=CARTESIAN_POINT('',(-2.46326859021798,-6.4,-1.13349364905389)) ;
#20910=CARTESIAN_POINT('Origin',(-2.21326859021798,-6.05,-1.56650635094611)) ;
#20911=CARTESIAN_POINT('',(-2.47307621135332,-6.4,-1.71650635094611)) ;
#20912=CARTESIAN_POINT('',(-2.21326859021798,-6.4,-1.56650635094611)) ;
#20913=CARTESIAN_POINT('',(-2.47307621135332,-6.05,-1.71650635094611)) ;
#20914=CARTESIAN_POINT('Origin',(-2.59807621135332,-6.05,-1.5)) ;
#20915=CARTESIAN_POINT('',(-2.59807621135332,-6.4,-1.5)) ;
#20916=CARTESIAN_POINT('Origin',(0.,-6.05,0.)) ;
#20917=CARTESIAN_POINT('',(-2.48746859276655,-6.4,-0.25)) ;
#20918=CARTESIAN_POINT('Origin',(0.,-6.4,0.)) ;
#20919=CARTESIAN_POINT('',(-2.48746859276655,-6.05,-0.25)) ;
#20920=CARTESIAN_POINT('Origin',(-2.7,-6.05,-0.25)) ;
#20921=CARTESIAN_POINT('',(-3.,-6.4,-0.25)) ;
#20922=CARTESIAN_POINT('',(-2.7,-6.4,-0.25)) ;
#20923=CARTESIAN_POINT('',(-3.,-6.05,-0.25)) ;
#20924=CARTESIAN_POINT('Origin',(-2.7,-6.05,0.25)) ;
#20925=CARTESIAN_POINT('',(-2.48746859276655,-6.4,0.25)) ;
#20926=CARTESIAN_POINT('',(-2.48746859276655,-6.05,0.25)) ;
#20927=CARTESIAN_POINT('',(-3.,-6.4,0.25)) ;
#20928=CARTESIAN_POINT('',(-3.,-6.05,0.25)) ;
#20929=CARTESIAN_POINT('',(-2.7,-6.4,0.25)) ;
#20930=CARTESIAN_POINT('Origin',(-3.,-6.05,3.67394039744206E-16)) ;
#20931=CARTESIAN_POINT('',(-3.,-6.4,3.67394039744206E-16)) ;
#20932=CARTESIAN_POINT('Origin',(0.,-6.05,0.)) ;
#20933=CARTESIAN_POINT('',(-2.27921099245176,-6.4,1.02722794543717)) ;
#20934=CARTESIAN_POINT('Origin',(0.,-6.4,0.)) ;
#20935=CARTESIAN_POINT('',(-2.27921099245176,-6.05,1.02722794543716)) ;
#20936=CARTESIAN_POINT('Origin',(-2.21326859021798,-6.05,1.56650635094611)) ;
#20937=CARTESIAN_POINT('',(-2.02921099245176,-6.4,1.46024064732938)) ;
#20938=CARTESIAN_POINT('',(-2.02921099245176,-6.05,1.46024064732938)) ;
#20939=CARTESIAN_POINT('',(-2.47307621135332,-6.4,1.71650635094611)) ;
#20940=CARTESIAN_POINT('',(-2.47307621135332,-6.05,1.71650635094611)) ;
#20941=CARTESIAN_POINT('',(-2.21326859021798,-6.4,1.56650635094611)) ;
#20942=CARTESIAN_POINT('Origin',(-2.46326859021798,-6.05,1.13349364905389)) ;
#20943=CARTESIAN_POINT('',(-2.72307621135332,-6.4,1.28349364905389)) ;
#20944=CARTESIAN_POINT('',(-2.46326859021798,-6.4,1.13349364905389)) ;
#20945=CARTESIAN_POINT('',(-2.72307621135332,-6.05,1.28349364905389)) ;
#20946=CARTESIAN_POINT('Origin',(-2.59807621135332,-6.05,1.5)) ;
#20947=CARTESIAN_POINT('',(-2.59807621135332,-6.4,1.5)) ;
#20948=CARTESIAN_POINT('Origin',(0.,-6.05,0.)) ;
#20949=CARTESIAN_POINT('',(-1.46024064732938,-6.4,2.02921099245176)) ;
#20950=CARTESIAN_POINT('Origin',(0.,-6.4,0.)) ;
#20951=CARTESIAN_POINT('',(-1.46024064732938,-6.05,2.02921099245176)) ;
#20952=CARTESIAN_POINT('Origin',(-1.56650635094611,-6.05,2.21326859021798)) ;
#20953=CARTESIAN_POINT('',(-1.71650635094611,-6.4,2.47307621135332)) ;
#20954=CARTESIAN_POINT('',(-1.56650635094611,-6.4,2.21326859021798)) ;
#20955=CARTESIAN_POINT('',(-1.71650635094611,-6.05,2.47307621135332)) ;
#20956=CARTESIAN_POINT('Origin',(-1.13349364905389,-6.05,2.46326859021798)) ;
#20957=CARTESIAN_POINT('',(-1.02722794543716,-6.4,2.27921099245176)) ;
#20958=CARTESIAN_POINT('',(-1.02722794543716,-6.05,2.27921099245176)) ;
#20959=CARTESIAN_POINT('',(-1.28349364905389,-6.4,2.72307621135332)) ;
#20960=CARTESIAN_POINT('',(-1.28349364905389,-6.05,2.72307621135332)) ;
#20961=CARTESIAN_POINT('',(-1.13349364905389,-6.4,2.46326859021798)) ;
#20962=CARTESIAN_POINT('Origin',(-1.5,-6.05,2.59807621135332)) ;
#20963=CARTESIAN_POINT('',(-1.5,-6.4,2.59807621135332)) ;
#20964=CARTESIAN_POINT('Origin',(0.,-6.05,0.)) ;
#20965=CARTESIAN_POINT('',(-0.25,-6.4,2.48746859276655)) ;
#20966=CARTESIAN_POINT('Origin',(0.,-6.4,0.)) ;
#20967=CARTESIAN_POINT('',(-0.25,-6.05,2.48746859276655)) ;
#20968=CARTESIAN_POINT('Origin',(0.25,-6.05,2.7)) ;
#20969=CARTESIAN_POINT('',(0.25,-6.4,2.48746859276655)) ;
#20970=CARTESIAN_POINT('',(0.25,-6.05,2.48746859276655)) ;
#20971=CARTESIAN_POINT('',(0.25,-6.4,3.)) ;
#20972=CARTESIAN_POINT('',(0.25,-6.05,3.)) ;
#20973=CARTESIAN_POINT('',(0.25,-6.4,2.7)) ;
#20974=CARTESIAN_POINT('Origin',(-0.25,-6.05,2.7)) ;
#20975=CARTESIAN_POINT('',(-0.25,-6.4,3.)) ;
#20976=CARTESIAN_POINT('',(-0.25,-6.4,2.7)) ;
#20977=CARTESIAN_POINT('',(-0.25,-6.05,3.)) ;
#20978=CARTESIAN_POINT('Origin',(1.83697019872103E-16,-6.05,3.)) ;
#20979=CARTESIAN_POINT('',(1.83697019872103E-16,-6.4,3.)) ;
#20980=CARTESIAN_POINT('Origin',(0.,-6.05,0.)) ;
#20981=CARTESIAN_POINT('',(1.02722794543717,-6.4,2.27921099245176)) ;
#20982=CARTESIAN_POINT('Origin',(0.,-6.4,0.)) ;
#20983=CARTESIAN_POINT('',(1.02722794543717,-6.05,2.27921099245176)) ;
#20984=CARTESIAN_POINT('Origin',(1.13349364905389,-6.05,2.46326859021798)) ;
#20985=CARTESIAN_POINT('',(1.28349364905389,-6.4,2.72307621135332)) ;
#20986=CARTESIAN_POINT('',(1.13349364905389,-6.4,2.46326859021798)) ;
#20987=CARTESIAN_POINT('',(1.28349364905389,-6.05,2.72307621135332)) ;
#20988=CARTESIAN_POINT('Origin',(1.56650635094611,-6.05,2.21326859021798)) ;
#20989=CARTESIAN_POINT('',(1.46024064732938,-6.4,2.02921099245176)) ;
#20990=CARTESIAN_POINT('',(1.46024064732938,-6.05,2.02921099245176)) ;
#20991=CARTESIAN_POINT('',(1.71650635094611,-6.4,2.47307621135332)) ;
#20992=CARTESIAN_POINT('',(1.71650635094611,-6.05,2.47307621135332)) ;
#20993=CARTESIAN_POINT('',(1.56650635094611,-6.4,2.21326859021798)) ;
#20994=CARTESIAN_POINT('Origin',(1.5,-6.05,2.59807621135332)) ;
#20995=CARTESIAN_POINT('',(1.5,-6.4,2.59807621135332)) ;
#20996=CARTESIAN_POINT('Origin',(0.,-6.05,0.)) ;
#20997=CARTESIAN_POINT('',(2.02921099245176,-6.4,1.46024064732938)) ;
#20998=CARTESIAN_POINT('Origin',(0.,-6.4,0.)) ;
#20999=CARTESIAN_POINT('',(2.02921099245176,-6.05,1.46024064732938)) ;
#21000=CARTESIAN_POINT('Origin',(2.46326859021798,-6.05,1.13349364905389)) ;
#21001=CARTESIAN_POINT('',(2.27921099245176,-6.4,1.02722794543717)) ;
#21002=CARTESIAN_POINT('',(2.27921099245176,-6.05,1.02722794543716)) ;
#21003=CARTESIAN_POINT('',(2.72307621135332,-6.4,1.28349364905389)) ;
#21004=CARTESIAN_POINT('',(2.72307621135332,-6.05,1.28349364905389)) ;
#21005=CARTESIAN_POINT('',(2.46326859021798,-6.4,1.13349364905389)) ;
#21006=CARTESIAN_POINT('Origin',(2.21326859021798,-6.05,1.56650635094611)) ;
#21007=CARTESIAN_POINT('',(2.47307621135332,-6.4,1.71650635094611)) ;
#21008=CARTESIAN_POINT('',(2.21326859021798,-6.4,1.56650635094611)) ;
#21009=CARTESIAN_POINT('',(2.47307621135332,-6.05,1.71650635094611)) ;
#21010=CARTESIAN_POINT('Origin',(2.59807621135332,-6.05,1.5)) ;
#21011=CARTESIAN_POINT('',(2.59807621135332,-6.4,1.5)) ;
#21012=CARTESIAN_POINT('Origin',(0.,-6.05,0.)) ;
#21013=CARTESIAN_POINT('',(2.48746859276655,-6.4,0.25)) ;
#21014=CARTESIAN_POINT('Origin',(0.,-6.4,0.)) ;
#21015=CARTESIAN_POINT('',(2.48746859276655,-6.05,0.25)) ;
#21016=CARTESIAN_POINT('Origin',(2.7,-6.05,0.25)) ;
#21017=CARTESIAN_POINT('',(3.,-6.4,0.25)) ;
#21018=CARTESIAN_POINT('',(2.7,-6.4,0.25)) ;
#21019=CARTESIAN_POINT('',(3.,-6.05,0.25)) ;
#21020=CARTESIAN_POINT('Origin',(2.7,-6.05,-0.25)) ;
#21021=CARTESIAN_POINT('',(3.,-6.4,-0.25)) ;
#21022=CARTESIAN_POINT('',(3.,-6.05,-0.25)) ;
#21023=CARTESIAN_POINT('',(2.7,-6.4,-0.25)) ;
#21024=CARTESIAN_POINT('Origin',(3.,-6.05,0.)) ;
#21025=CARTESIAN_POINT('',(3.,-6.4,0.)) ;
#21026=CARTESIAN_POINT('Origin',(0.,-6.25,0.)) ;
#21027=CARTESIAN_POINT('',(-1.4,-6.4,1.71450551880629E-16)) ;
#21028=CARTESIAN_POINT('Origin',(0.,-6.4,0.)) ;
#21029=CARTESIAN_POINT('',(-1.4,-6.25,1.71450551880629E-16)) ;
#21030=CARTESIAN_POINT('Origin',(0.,-6.4,0.)) ;
#24545=UNCERTAINTY_MEASURE_WITH_UNIT(LENGTH_MEASURE(0.001),#24629,
'DISTANCE_ACCURACY_VALUE',
'Maximum model space distance between geometric entities at asserted c
onnectivities') ;
#24580=UNCERTAINTY_MEASURE_WITH_UNIT(LENGTH_MEASURE(0.001),#24629,
'DISTANCE_ACCURACY_VALUE',
'Maximum model space distance between geometric entities at asserted c
onnectivities') ;
#24593=(
GEOMETRIC_REPRESENTATION_CONTEXT(3)
GLOBAL_UNCERTAINTY_ASSIGNED_CONTEXT((#24545))
GLOBAL_UNIT_ASSIGNED_CONTEXT((#24629,#24631,#24632))
REPRESENTATION_CONTEXT('','3D')
) ;
#24628=(
GEOMETRIC_REPRESENTATION_CONTEXT(3)
GLOBAL_UNCERTAINTY_ASSIGNED_CONTEXT((#24580))
GLOBAL_UNIT_ASSIGNED_CONTEXT((#24629,#24631,#24632))
REPRESENTATION_CONTEXT('','3D')
) ;
#24629=(
LENGTH_UNIT()
NAMED_UNIT(*)
SI_UNIT(.CENTI.,.METRE.)
) ;
#24631=(
NAMED_UNIT(*)
PLANE_ANGLE_UNIT()
SI_UNIT($,.RADIAN.)
) ;
#24632=(
NAMED_UNIT(*)
SI_UNIT($,.STERADIAN.)
SOLID_ANGLE_UNIT()
) ;
#24645=SHAPE_DEFINITION_REPRESENTATION(#24692,#24803) ;
#24692=PRODUCT_DEFINITION_SHAPE('',$,#24851) ;
#24803=SHAPE_REPRESENTATION('',(#14115),#24593) ;
#24838=PRODUCT_DEFINITION_CONTEXT('part definition',#24981,'design') ;
#24851=PRODUCT_DEFINITION('DRIVE_SPROCKET_12T',
'DRIVE_SPROCKET_12T',#24898,#24838) ;
#24898=PRODUCT_DEFINITION_FORMATION('',$,#24995) ;
#24981=APPLICATION_CONTEXT(
'Core Data for Automotive Mechanical Design Process') ;
#24982=PRODUCT_CONTEXT('part definition',#24981,'mechanical') ;
#24995=PRODUCT('DRIVE_SPROCKET_12T','DRIVE_SPROCKET_12T',$,(#24982)) ;
#25030=PRESENTATION_STYLE_ASSIGNMENT((#25040)) ;
#25040=SURFACE_STYLE_USAGE(.BOTH.,#25050) ;
#25050=SURFACE_SIDE_STYLE('',(#25060)) ;
#25060=SURFACE_STYLE_FILL_AREA(#25070) ;
#25070=FILL_AREA_STYLE('Steel - Satin',(#25080)) ;
#25080=FILL_AREA_STYLE_COLOUR('Steel - Satin',#25090) ;
#25090=COLOUR_RGB('Steel - Satin', 0.66274510, 0.83137255, 0.94901961) ;
ENDSEC;
END-ISO-10303-21;
